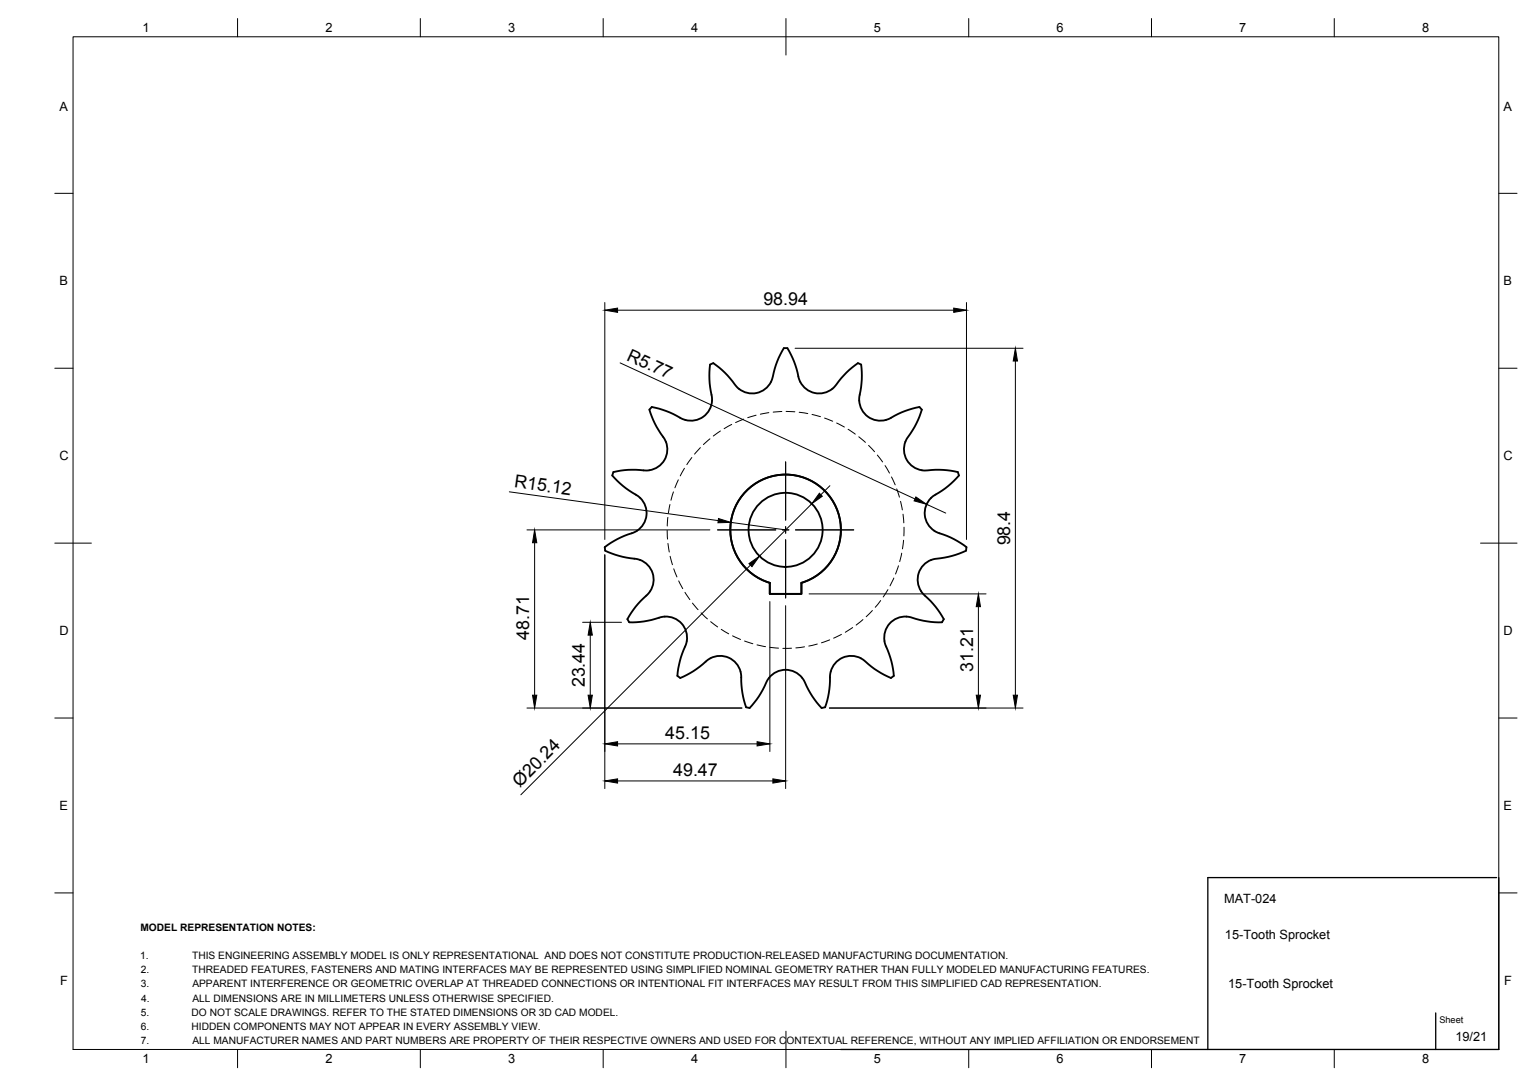
ISO-10303-21;
HEADER;
/* Generated by software containing ST-Developer
 * from STEP Tools, Inc. (www.steptools.com) 
 */

FILE_DESCRIPTION(
/* description */ ('STEP AP214'),
/* implementation_level */ '2;1');

FILE_NAME(
/* name */ '15-Tooth Sprocket.step',
/* time_stamp */ '2026-11-14T06:34:07-08:00',
/* author */ (''),
/* organization */ (''),
/* preprocessor_version */ 'ST-DEVELOPER v20.2',
/* originating_system */ 'Autodesk Translation Framework v15.17.0.0',
/* authorisation */ '');

FILE_SCHEMA (('AUTOMOTIVE_DESIGN { 1 0 10303 214 3 1 1 }'));
ENDSEC;

DATA;
#10=MECHANICAL_DESIGN_GEOMETRIC_PRESENTATION_REPRESENTATION('',(#7279,#7280),#310623);
#4024=TOROIDAL_SURFACE('',#103341,32.976,0.576);
#4025=TOROIDAL_SURFACE('',#103396,40.6764810164406,18.288);
#4026=TOROIDAL_SURFACE('',#103398,40.6764810164406,18.288);
#4027=TOROIDAL_SURFACE('',#103400,40.6764810164406,18.288);
#4028=TOROIDAL_SURFACE('',#103402,40.6764810164406,18.288);
#4029=TOROIDAL_SURFACE('',#103404,40.6764810164406,18.288);
#4030=TOROIDAL_SURFACE('',#103406,40.6764810164406,18.288);
#4031=TOROIDAL_SURFACE('',#103408,40.6764810164406,18.288);
#4032=TOROIDAL_SURFACE('',#103410,40.6764810164406,18.288);
#4033=TOROIDAL_SURFACE('',#103412,40.6764810164406,18.288);
#4034=TOROIDAL_SURFACE('',#103414,40.6764810164406,18.288);
#4035=TOROIDAL_SURFACE('',#103416,40.6764810164406,18.288);
#4036=TOROIDAL_SURFACE('',#103418,40.6764810164406,18.288);
#4037=TOROIDAL_SURFACE('',#103420,40.6764810164406,18.288);
#4038=TOROIDAL_SURFACE('',#103422,40.6764810164406,18.288);
#4039=TOROIDAL_SURFACE('',#103452,40.6764810164406,18.288);
#4040=TOROIDAL_SURFACE('',#103454,40.6764810164406,18.288);
#4041=TOROIDAL_SURFACE('',#103456,40.6764810164406,18.288);
#4042=TOROIDAL_SURFACE('',#103458,40.6764810164406,18.288);
#4043=TOROIDAL_SURFACE('',#103460,40.6764810164406,18.288);
#4044=TOROIDAL_SURFACE('',#103462,40.6764810164406,18.288);
#4045=TOROIDAL_SURFACE('',#103464,40.6764810164406,18.288);
#4046=TOROIDAL_SURFACE('',#103466,40.6764810164406,18.288);
#4047=TOROIDAL_SURFACE('',#103468,40.6764810164406,18.288);
#4048=TOROIDAL_SURFACE('',#103470,40.6764810164406,18.288);
#4049=TOROIDAL_SURFACE('',#103472,40.6764810164406,18.288);
#4050=TOROIDAL_SURFACE('',#103474,40.6764810164406,18.288);
#4051=TOROIDAL_SURFACE('',#103476,40.6764810164406,18.288);
#4052=TOROIDAL_SURFACE('',#103478,40.6764810164406,18.288);
#4053=TOROIDAL_SURFACE('',#103480,40.6764810164406,18.288);
#4054=TOROIDAL_SURFACE('',#103484,40.6764810164406,18.288);
#6306=B_SPLINE_CURVE_WITH_KNOTS('',3,(#271237,#271238,#271239,#271240,#271241,
#271242,#271243,#271244),.UNSPECIFIED.,.F.,.F.,(4,2,2,4),(-8.98049293427854,
-8.97889171867458,-8.34884827602697,-8.12983481855878),.UNSPECIFIED.);
#6307=B_SPLINE_CURVE_WITH_KNOTS('',3,(#271248,#271249,#271250,#271251,#271252,
#271253),.UNSPECIFIED.,.F.,.F.,(4,2,4),(-2.68771546706156,-2.29799156778152,
-1.97285776109994),.UNSPECIFIED.);
#6308=B_SPLINE_CURVE_WITH_KNOTS('',3,(#271258,#271259,#271260,#271261,#271262,
#271263),.UNSPECIFIED.,.F.,.F.,(4,2,4),(0.518273427329016,0.647448708132802,
0.677306880099543),.UNSPECIFIED.);
#6309=B_SPLINE_CURVE_WITH_KNOTS('',3,(#271267,#271268,#271269,#271270),
 .UNSPECIFIED.,.F.,.F.,(4,4),(1.16920248436213,1.3284621703947),
 .UNSPECIFIED.);
#6310=B_SPLINE_CURVE_WITH_KNOTS('',3,(#271274,#271275,#271276,#271277,#271278,
#271279),.UNSPECIFIED.,.F.,.F.,(4,2,4),(2.36444145730686,2.40335316097516,
2.52343865872206),.UNSPECIFIED.);
#6311=B_SPLINE_CURVE_WITH_KNOTS('',3,(#271283,#271284,#271285,#271286,#271287,
#271288),.UNSPECIFIED.,.F.,.F.,(4,2,4),(3.01719559991105,3.07732160469005,
3.17624638273508),.UNSPECIFIED.);
#6312=B_SPLINE_CURVE_WITH_KNOTS('',3,(#271295,#271296,#271297,#271298,#271299,
#271300),.UNSPECIFIED.,.F.,.F.,(4,2,4),(0.51827342732949,0.647448708132718,
0.677306880099455),.UNSPECIFIED.);
#6313=B_SPLINE_CURVE_WITH_KNOTS('',3,(#271304,#271305,#271306,#271307),
 .UNSPECIFIED.,.F.,.F.,(4,4),(1.16920248460095,1.3284621706712),
 .UNSPECIFIED.);
#6314=B_SPLINE_CURVE_WITH_KNOTS('',3,(#271311,#271312,#271313,#271314,#271315,
#271316),.UNSPECIFIED.,.F.,.F.,(4,2,4),(2.36444145785531,2.40335316153482,
2.5234386593167),.UNSPECIFIED.);
#6315=B_SPLINE_CURVE_WITH_KNOTS('',3,(#271319,#271320,#271321,#271322,#271323,
#271324),.UNSPECIFIED.,.F.,.F.,(4,2,4),(3.01719559991067,3.07732160468965,
3.17624638273467),.UNSPECIFIED.);
#6316=B_SPLINE_CURVE_WITH_KNOTS('',3,(#271330,#271331,#271332,#271333,#271334,
#271335),.UNSPECIFIED.,.F.,.F.,(4,2,4),(0.51827342732973,0.647448708133012,
0.677306880099766),.UNSPECIFIED.);
#6317=B_SPLINE_CURVE_WITH_KNOTS('',3,(#271339,#271340,#271341,#271342),
 .UNSPECIFIED.,.F.,.F.,(4,4),(1.16920248436227,1.32846217039502),
 .UNSPECIFIED.);
#6318=B_SPLINE_CURVE_WITH_KNOTS('',3,(#271346,#271347,#271348,#271349,#271350,
#271351),.UNSPECIFIED.,.F.,.F.,(4,2,4),(2.36444145730766,2.40335316097597,
2.523438658723),.UNSPECIFIED.);
#6319=B_SPLINE_CURVE_WITH_KNOTS('',3,(#271354,#271355,#271356,#271357,#271358,
#271359),.UNSPECIFIED.,.F.,.F.,(4,2,4),(3.0171955999124,3.07732160469143,
3.1762463827365),.UNSPECIFIED.);
#6320=B_SPLINE_CURVE_WITH_KNOTS('',3,(#271363,#271364,#271365,#271366,#271367,
#271368),.UNSPECIFIED.,.F.,.F.,(4,2,4),(3.01719559991218,3.07732160469121,
3.17624638273563),.UNSPECIFIED.);
#6321=B_SPLINE_CURVE_WITH_KNOTS('',3,(#271372,#271373,#271374,#271375,#271376,
#271377),.UNSPECIFIED.,.F.,.F.,(4,2,4),(0.518273427329665,0.647448708132928,
0.677306880099671),.UNSPECIFIED.);
#6322=B_SPLINE_CURVE_WITH_KNOTS('',3,(#271381,#271382,#271383,#271384),
 .UNSPECIFIED.,.F.,.F.,(4,4),(1.1692024843613,1.32846217039385),
 .UNSPECIFIED.);
#6323=B_SPLINE_CURVE_WITH_KNOTS('',3,(#271388,#271389,#271390,#271391,#271392,
#271393),.UNSPECIFIED.,.F.,.F.,(4,2,4),(2.36444145730499,2.40335316097287,
2.52343865871962),.UNSPECIFIED.);
#6324=B_SPLINE_CURVE_WITH_KNOTS('',3,(#271400,#271401,#271402,#271403,#271404,
#271405),.UNSPECIFIED.,.F.,.F.,(4,2,4),(0.518273427329571,0.647448708132802,
0.677306880099541),.UNSPECIFIED.);
#6325=B_SPLINE_CURVE_WITH_KNOTS('',3,(#271409,#271410,#271411,#271412),
 .UNSPECIFIED.,.F.,.F.,(4,4),(1.16920248412223,1.32846217011725),
 .UNSPECIFIED.);
#6326=B_SPLINE_CURVE_WITH_KNOTS('',3,(#271416,#271417,#271418,#271419,#271420,
#271421),.UNSPECIFIED.,.F.,.F.,(4,2,4),(2.3644414567562,2.40335316041326,
2.52343865812509),.UNSPECIFIED.);
#6327=B_SPLINE_CURVE_WITH_KNOTS('',3,(#271424,#271425,#271426,#271427,#271428,
#271429),.UNSPECIFIED.,.F.,.F.,(4,2,4),(3.01719559991075,3.07732160468976,
3.17624638273476),.UNSPECIFIED.);
#6328=B_SPLINE_CURVE_WITH_KNOTS('',3,(#271435,#271436,#271437,#271438,#271439,
#271440),.UNSPECIFIED.,.F.,.F.,(4,2,4),(0.518273427329574,0.647448708132822,
0.677306880099564),.UNSPECIFIED.);
#6329=B_SPLINE_CURVE_WITH_KNOTS('',3,(#271444,#271445,#271446,#271447),
 .UNSPECIFIED.,.F.,.F.,(4,4),(1.16920248436231,1.32846217039508),
 .UNSPECIFIED.);
#6330=B_SPLINE_CURVE_WITH_KNOTS('',3,(#271451,#271452,#271453,#271454,#271455,
#271456),.UNSPECIFIED.,.F.,.F.,(4,2,4),(2.3644414573074,2.40335316097572,
2.52343865872264),.UNSPECIFIED.);
#6331=B_SPLINE_CURVE_WITH_KNOTS('',3,(#271459,#271460,#271461,#271462,#271463,
#271464),.UNSPECIFIED.,.F.,.F.,(4,2,4),(3.01719559991156,3.07732160469059,
3.17624638273566),.UNSPECIFIED.);
#6332=B_SPLINE_CURVE_WITH_KNOTS('',3,(#271468,#271469,#271470,#271471,#271472,
#271473),.UNSPECIFIED.,.F.,.F.,(4,2,4),(-2.68771546706066,-2.29799156778083,
-1.9728577610994),.UNSPECIFIED.);
#6333=B_SPLINE_CURVE_WITH_KNOTS('',3,(#271477,#271478,#271479,#271480,#271481,
#271482,#271483,#271484),.UNSPECIFIED.,.F.,.F.,(4,2,2,4),(-8.98049293427925,
-8.97889171867529,-8.34884827602781,-8.12983481855968),.UNSPECIFIED.);
#6334=B_SPLINE_CURVE_WITH_KNOTS('',3,(#271552,#271553,#271554,#271555,#271556,
#271557,#271558,#271559),.UNSPECIFIED.,.F.,.F.,(4,2,2,4),(-8.98049293427854,
-8.97889171867458,-8.34884827602725,-8.12983481855919),.UNSPECIFIED.);
#6335=B_SPLINE_CURVE_WITH_KNOTS('',3,(#271563,#271564,#271565,#271566,#271567,
#271568),.UNSPECIFIED.,.F.,.F.,(4,2,4),(-2.68771546706143,-2.29799156778143,
-1.97285776109989),.UNSPECIFIED.);
#6336=B_SPLINE_CURVE_WITH_KNOTS('',3,(#271569,#271570,#271571,#271572,#271573,
#271574),.UNSPECIFIED.,.F.,.F.,(4,2,4),(0.51827342732961,0.64744870813287,
0.677306880099612),.UNSPECIFIED.);
#6337=B_SPLINE_CURVE_WITH_KNOTS('',3,(#271575,#271576,#271577,#271578,#271579,
#271580),.UNSPECIFIED.,.F.,.F.,(4,2,4),(3.0171955999114,3.07732160469042,
3.17624638273548),.UNSPECIFIED.);
#6338=B_SPLINE_CURVE_WITH_KNOTS('',3,(#271583,#271584,#271585,#271586,#271587,
#271588),.UNSPECIFIED.,.F.,.F.,(4,2,4),(0.518273427329597,0.647448708132832,
0.677306880099573),.UNSPECIFIED.);
#6339=B_SPLINE_CURVE_WITH_KNOTS('',3,(#271590,#271591,#271592,#271593,#271594,
#271595),.UNSPECIFIED.,.F.,.F.,(4,2,4),(3.01719559990933,3.07732160468829,
3.17624638273323),.UNSPECIFIED.);
#6340=B_SPLINE_CURVE_WITH_KNOTS('',3,(#271597,#271598,#271599,#271600,#271601,
#271602,#271603,#271604),.UNSPECIFIED.,.F.,.F.,(4,2,2,4),(-8.98049293427795,
-8.97889171867398,-8.3488482760265,-8.12983481855838),.UNSPECIFIED.);
#6341=B_SPLINE_CURVE_WITH_KNOTS('',3,(#271607,#271608,#271609,#271610,#271611,
#271612),.UNSPECIFIED.,.F.,.F.,(4,2,4),(-2.6877154670615,-2.29799156778146,
-1.97285776109988),.UNSPECIFIED.);
#6342=B_SPLINE_CURVE_WITH_KNOTS('',3,(#271615,#271616,#271617,#271618,#271619,
#271620),.UNSPECIFIED.,.F.,.F.,(4,2,4),(0.518273427329312,0.647448708132468,
0.677306880099178),.UNSPECIFIED.);
#6343=B_SPLINE_CURVE_WITH_KNOTS('',3,(#271622,#271623,#271624,#271625,#271626,
#271627),.UNSPECIFIED.,.F.,.F.,(4,2,4),(3.0171955999108,3.0773216046898,
3.1762463827348),.UNSPECIFIED.);
#6344=B_SPLINE_CURVE_WITH_KNOTS('',3,(#271629,#271630,#271631,#271632,#271633,
#271634,#271635,#271636),.UNSPECIFIED.,.F.,.F.,(4,2,2,4),(-8.98049293427752,
-8.97889171867356,-8.34884827602617,-8.12983481855807),.UNSPECIFIED.);
#6345=B_SPLINE_CURVE_WITH_KNOTS('',3,(#271639,#271640,#271641,#271642,#271643,
#271644),.UNSPECIFIED.,.F.,.F.,(4,2,4),(-2.68771546706155,-2.29799156778148,
-1.9728577610999),.UNSPECIFIED.);
#6346=B_SPLINE_CURVE_WITH_KNOTS('',3,(#271647,#271648,#271649,#271650,#271651,
#271652),.UNSPECIFIED.,.F.,.F.,(4,2,4),(0.518273427329541,0.647448708132767,
0.6773068800995),.UNSPECIFIED.);
#6347=B_SPLINE_CURVE_WITH_KNOTS('',3,(#271654,#271655,#271656,#271657,#271658,
#271659),.UNSPECIFIED.,.F.,.F.,(4,2,4),(3.01719559991074,3.07732160468976,
3.17624638273482),.UNSPECIFIED.);
#6348=B_SPLINE_CURVE_WITH_KNOTS('',3,(#271661,#271662,#271663,#271664,#271665,
#271666,#271667,#271668),.UNSPECIFIED.,.F.,.F.,(4,2,2,4),(-8.98049293427772,
-8.97889171867376,-8.34884827602598,-8.12983481855773),.UNSPECIFIED.);
#6349=B_SPLINE_CURVE_WITH_KNOTS('',3,(#271671,#271672,#271673,#271674,#271675,
#271676),.UNSPECIFIED.,.F.,.F.,(4,2,4),(-2.68771546706066,-2.29799156778086,
-1.97285776109946),.UNSPECIFIED.);
#6350=B_SPLINE_CURVE_WITH_KNOTS('',3,(#271681,#271682,#271683,#271684,#271685,
#271686),.UNSPECIFIED.,.F.,.F.,(4,2,4),(-2.68771546706142,-2.29799156778141,
-1.97285776109986),.UNSPECIFIED.);
#6351=B_SPLINE_CURVE_WITH_KNOTS('',3,(#271687,#271688,#271689,#271690,#271691,
#271692),.UNSPECIFIED.,.F.,.F.,(4,2,4),(0.518273427329233,0.647448708132411,
0.677306880099119),.UNSPECIFIED.);
#6352=B_SPLINE_CURVE_WITH_KNOTS('',3,(#271693,#271694,#271695,#271696,#271697,
#271698),.UNSPECIFIED.,.F.,.F.,(4,2,4),(3.01719559991029,3.0773216046893,
3.17624638273431),.UNSPECIFIED.);
#6353=B_SPLINE_CURVE_WITH_KNOTS('',3,(#271701,#271702,#271703,#271704,#271705,
#271706),.UNSPECIFIED.,.F.,.F.,(4,2,4),(0.518273427329369,0.647448708132555,
0.677306880099271),.UNSPECIFIED.);
#6354=B_SPLINE_CURVE_WITH_KNOTS('',3,(#271708,#271709,#271710,#271711,#271712,
#271713),.UNSPECIFIED.,.F.,.F.,(4,2,4),(3.01719559991216,3.07732160469119,
3.17624638273627),.UNSPECIFIED.);
#6355=B_SPLINE_CURVE_WITH_KNOTS('',3,(#271715,#271716,#271717,#271718,#271719,
#271720,#271721,#271722),.UNSPECIFIED.,.F.,.F.,(4,2,2,4),(-8.98049293427722,
-8.97889171867326,-8.34884827602583,-8.1298348185577),.UNSPECIFIED.);
#6356=B_SPLINE_CURVE_WITH_KNOTS('',3,(#271725,#271726,#271727,#271728,#271729,
#271730),.UNSPECIFIED.,.F.,.F.,(4,2,4),(-2.68771546706111,-2.29799156778117,
-1.97285776109968),.UNSPECIFIED.);
#6357=B_SPLINE_CURVE_WITH_KNOTS('',3,(#271734,#271735,#271736,#271737,#271738,
#271739,#271740,#271741),.UNSPECIFIED.,.F.,.F.,(4,2,2,4),(-8.98049293427961,
-8.97889171867565,-8.34884827602804,-8.12983481855986),.UNSPECIFIED.);
#6358=B_SPLINE_CURVE_WITH_KNOTS('',3,(#271745,#271746,#271747,#271748,#271749,
#271750),.UNSPECIFIED.,.F.,.F.,(4,2,4),(-2.68771546706186,-2.29799156778171,
-1.97285776110007),.UNSPECIFIED.);
#6359=B_SPLINE_CURVE_WITH_KNOTS('',3,(#271751,#271752,#271753,#271754,#271755,
#271756),.UNSPECIFIED.,.F.,.F.,(4,2,4),(0.51827342732934,0.647448708132526,
0.677306880099254),.UNSPECIFIED.);
#6360=B_SPLINE_CURVE_WITH_KNOTS('',3,(#271757,#271758,#271759,#271760,#271761,
#271762),.UNSPECIFIED.,.F.,.F.,(4,2,4),(3.01719559990916,3.07732160468812,
3.17624638273306),.UNSPECIFIED.);
#6361=B_SPLINE_CURVE_WITH_KNOTS('',3,(#271765,#271766,#271767,#271768,#271769,
#271770,#271771,#271772),.UNSPECIFIED.,.F.,.F.,(4,2,2,4),(-8.98049293427778,
-8.97889171867381,-8.34884827602637,-8.12983481855824),.UNSPECIFIED.);
#6362=B_SPLINE_CURVE_WITH_KNOTS('',3,(#271775,#271776,#271777,#271778,#271779,
#271780),.UNSPECIFIED.,.F.,.F.,(4,2,4),(-2.68771546706139,-2.29799156778137,
-1.97285776109982),.UNSPECIFIED.);
#6363=B_SPLINE_CURVE_WITH_KNOTS('',3,(#271783,#271784,#271785,#271786,#271787,
#271788),.UNSPECIFIED.,.F.,.F.,(4,2,4),(3.01719559990971,3.07732160468868,
3.17624638273366),.UNSPECIFIED.);
#6364=B_SPLINE_CURVE_WITH_KNOTS('',3,(#271790,#271791,#271792,#271793,#271794,
#271795,#271796,#271797),.UNSPECIFIED.,.F.,.F.,(4,2,2,4),(-8.98049293427817,
-8.97889171867421,-8.34884827602685,-8.12983481855876),.UNSPECIFIED.);
#6365=B_SPLINE_CURVE_WITH_KNOTS('',3,(#271800,#271801,#271802,#271803,#271804,
#271805),.UNSPECIFIED.,.F.,.F.,(4,2,4),(-2.68771546706148,-2.29799156778145,
-1.97285776109989),.UNSPECIFIED.);
#6366=B_SPLINE_CURVE_WITH_KNOTS('',3,(#271808,#271809,#271810,#271811,#271812,
#271813,#271814,#271815),.UNSPECIFIED.,.F.,.F.,(4,2,2,4),(-8.98049293427992,
-8.97889171867596,-8.34884827602816,-8.12983481855992),.UNSPECIFIED.);
#6367=B_SPLINE_CURVE_WITH_KNOTS('',3,(#271818,#271819,#271820,#271821,#271822,
#271823),.UNSPECIFIED.,.F.,.F.,(4,2,4),(-2.68771546706129,-2.29799156778129,
-1.97285776109976),.UNSPECIFIED.);
#6368=B_SPLINE_CURVE_WITH_KNOTS('',3,(#271826,#271827,#271828,#271829,#271830,
#271831,#271832,#271833),.UNSPECIFIED.,.F.,.F.,(4,2,2,4),(-8.98049293428024,
-8.97889171867627,-8.34884827602869,-8.12983481856052),.UNSPECIFIED.);
#6369=B_SPLINE_CURVE_WITH_KNOTS('',3,(#271836,#271837,#271838,#271839,#271840,
#271841),.UNSPECIFIED.,.F.,.F.,(4,2,4),(-2.68771546706172,-2.29799156778164,
-1.97285776110006),.UNSPECIFIED.);
#6370=B_SPLINE_CURVE_WITH_KNOTS('',3,(#271844,#271845,#271846,#271847,#271848,
#271849,#271850,#271851),.UNSPECIFIED.,.F.,.F.,(4,2,2,4),(-8.98049293427857,
-8.97889171867461,-8.34884827602675,-8.12983481855846),.UNSPECIFIED.);
#6371=B_SPLINE_CURVE_WITH_KNOTS('',3,(#271854,#271855,#271856,#271857,#271858,
#271859),.UNSPECIFIED.,.F.,.F.,(4,2,4),(-2.68771546706135,-2.29799156778136,
-1.97285776109983),.UNSPECIFIED.);
#6372=B_SPLINE_CURVE_WITH_KNOTS('',3,(#271862,#271863,#271864,#271865,#271866,
#271867,#271868,#271869),.UNSPECIFIED.,.F.,.F.,(4,2,2,4),(-8.98049293428122,
-8.97889171867726,-8.34884827602979,-8.12983481856169),.UNSPECIFIED.);
#6373=B_SPLINE_CURVE_WITH_KNOTS('',3,(#271873,#271874,#271875,#271876,#271877,
#271878),.UNSPECIFIED.,.F.,.F.,(4,2,4),(-2.68771546706168,-2.29799156778158,
-1.97285776109999),.UNSPECIFIED.);
#6374=B_SPLINE_CURVE_WITH_KNOTS('',3,(#271879,#271880,#271881,#271882,#271883,
#271884),.UNSPECIFIED.,.F.,.F.,(4,2,4),(0.518273427329314,0.647448708132495,
0.677306880099206),.UNSPECIFIED.);
#6375=B_SPLINE_CURVE_WITH_KNOTS('',3,(#271887,#271888,#271889,#271890,#271891,
#271892,#271893,#271894),.UNSPECIFIED.,.F.,.F.,(4,2,2,4),(-8.98049293427992,
-8.97889171867595,-8.34884827602839,-8.12983481856025),.UNSPECIFIED.);
#6376=B_SPLINE_CURVE_WITH_KNOTS('',3,(#271897,#271898,#271899,#271900,#271901,
#271902),.UNSPECIFIED.,.F.,.F.,(4,2,4),(-2.68771546706109,-2.29799156778117,
-1.97285776109969),.UNSPECIFIED.);
#6377=B_SPLINE_CURVE_WITH_KNOTS('',3,(#271987,#271988,#271989,#271990,#271991,
#271992),.UNSPECIFIED.,.F.,.F.,(4,2,4),(-2.68771546706178,-2.29799156778168,
-1.97285776110008),.UNSPECIFIED.);
#6378=B_SPLINE_CURVE_WITH_KNOTS('',3,(#271994,#271995,#271996,#271997,#271998,
#271999),.UNSPECIFIED.,.F.,.F.,(4,2,4),(2.36444145730966,2.403353160978,
2.52343865872509),.UNSPECIFIED.);
#6379=B_SPLINE_CURVE_WITH_KNOTS('',3,(#272003,#272004,#272005,#272006),
 .UNSPECIFIED.,.F.,.F.,(4,4),(1.16920248436245,1.32846217039523),
 .UNSPECIFIED.);
#6380=B_SPLINE_CURVE_WITH_KNOTS('',3,(#272007,#272008,#272009,#272010,#272011,
#272012,#272013,#272014),.UNSPECIFIED.,.F.,.F.,(4,2,2,4),(-8.98049293428071,
-8.97889171867675,-8.34884827602921,-8.12983481856106),.UNSPECIFIED.);
#6381=B_SPLINE_CURVE_WITH_KNOTS('',3,(#272018,#272019,#272020,#272021),
 .UNSPECIFIED.,.F.,.F.,(4,4),(1.16920248436348,1.32846217039639),
 .UNSPECIFIED.);
#6382=B_SPLINE_CURVE_WITH_KNOTS('',3,(#272022,#272023,#272024,#272025,#272026,
#272027,#272028,#272029),.UNSPECIFIED.,.F.,.F.,(4,2,2,4),(-8.98049293427966,
-8.97889171867569,-8.34884827602823,-8.12983481856012),.UNSPECIFIED.);
#6383=B_SPLINE_CURVE_WITH_KNOTS('',3,(#272031,#272032,#272033,#272034,#272035,
#272036),.UNSPECIFIED.,.F.,.F.,(4,2,4),(-2.68771546706079,-2.29799156778091,
-1.97285776109946),.UNSPECIFIED.);
#6384=B_SPLINE_CURVE_WITH_KNOTS('',3,(#272038,#272039,#272040,#272041,#272042,
#272043),.UNSPECIFIED.,.F.,.F.,(4,2,4),(2.36444145731017,2.40335316097854,
2.52343865872566),.UNSPECIFIED.);
#6385=B_SPLINE_CURVE_WITH_KNOTS('',3,(#272048,#272049,#272050,#272051),
 .UNSPECIFIED.,.F.,.F.,(4,4),(1.16920248436344,1.32846217039637),
 .UNSPECIFIED.);
#6386=B_SPLINE_CURVE_WITH_KNOTS('',3,(#272052,#272053,#272054,#272055,#272056,
#272057,#272058,#272059),.UNSPECIFIED.,.F.,.F.,(4,2,2,4),(-8.98049293427945,
-8.97889171867549,-8.34884827602783,-8.12983481855963),.UNSPECIFIED.);
#6387=B_SPLINE_CURVE_WITH_KNOTS('',3,(#272061,#272062,#272063,#272064,#272065,
#272066),.UNSPECIFIED.,.F.,.F.,(4,2,4),(-2.68771546706122,-2.29799156778128,
-1.97285776109977),.UNSPECIFIED.);
#6388=B_SPLINE_CURVE_WITH_KNOTS('',3,(#272068,#272069,#272070,#272071,#272072,
#272073),.UNSPECIFIED.,.F.,.F.,(4,2,4),(2.36444145675313,2.40335316041008,
2.52343865812168),.UNSPECIFIED.);
#6389=B_SPLINE_CURVE_WITH_KNOTS('',3,(#272078,#272079,#272080,#272081),
 .UNSPECIFIED.,.F.,.F.,(4,4),(1.16920248412103,1.32846217011589),
 .UNSPECIFIED.);
#6390=B_SPLINE_CURVE_WITH_KNOTS('',3,(#272082,#272083,#272084,#272085,#272086,
#272087,#272088,#272089),.UNSPECIFIED.,.F.,.F.,(4,2,2,4),(-8.98049293427762,
-8.97889171867365,-8.34884827602598,-8.12983481855776),.UNSPECIFIED.);
#6391=B_SPLINE_CURVE_WITH_KNOTS('',3,(#272091,#272092,#272093,#272094,#272095,
#272096),.UNSPECIFIED.,.F.,.F.,(4,2,4),(-2.68771546706239,-2.29799156778215,
-1.97285776110044),.UNSPECIFIED.);
#6392=B_SPLINE_CURVE_WITH_KNOTS('',3,(#272098,#272099,#272100,#272101,#272102,
#272103),.UNSPECIFIED.,.F.,.F.,(4,2,4),(2.36444145730695,2.40335316097526,
2.5234386587222),.UNSPECIFIED.);
#6393=B_SPLINE_CURVE_WITH_KNOTS('',3,(#272107,#272108,#272109,#272110,#272111,
#272112),.UNSPECIFIED.,.F.,.F.,(4,2,4),(2.36444145785125,2.4033531615307,
2.52343865931237),.UNSPECIFIED.);
#6394=B_SPLINE_CURVE_WITH_KNOTS('',3,(#272116,#272117,#272118,#272119),
 .UNSPECIFIED.,.F.,.F.,(4,4),(1.16920248436207,1.3284621703948),
 .UNSPECIFIED.);
#6395=B_SPLINE_CURVE_WITH_KNOTS('',3,(#272120,#272121,#272122,#272123,#272124,
#272125,#272126,#272127),.UNSPECIFIED.,.F.,.F.,(4,2,2,4),(-8.98049293427944,
-8.97889171867548,-8.34884827602771,-8.12983481855948),.UNSPECIFIED.);
#6396=B_SPLINE_CURVE_WITH_KNOTS('',3,(#272131,#272132,#272133,#272134),
 .UNSPECIFIED.,.F.,.F.,(4,4),(1.16920248459907,1.32846217066903),
 .UNSPECIFIED.);
#6397=B_SPLINE_CURVE_WITH_KNOTS('',3,(#272135,#272136,#272137,#272138,#272139,
#272140,#272141,#272142),.UNSPECIFIED.,.F.,.F.,(4,2,2,4),(-8.98049293428055,
-8.97889171867659,-8.34884827602886,-8.12983481856065),.UNSPECIFIED.);
#6398=B_SPLINE_CURVE_WITH_KNOTS('',3,(#272144,#272145,#272146,#272147,#272148,
#272149),.UNSPECIFIED.,.F.,.F.,(4,2,4),(-2.68771546706087,-2.297991567781,
-1.97285776109955),.UNSPECIFIED.);
#6399=B_SPLINE_CURVE_WITH_KNOTS('',3,(#272151,#272152,#272153,#272154,#272155,
#272156),.UNSPECIFIED.,.F.,.F.,(4,2,4),(2.36444145730775,2.4033531609761,
2.5234386587231),.UNSPECIFIED.);
#6400=B_SPLINE_CURVE_WITH_KNOTS('',3,(#272160,#272161,#272162,#272163,#272164,
#272165),.UNSPECIFIED.,.F.,.F.,(4,2,4),(-2.68771546706131,-2.29799156778135,
-1.97285776109984),.UNSPECIFIED.);
#6401=B_SPLINE_CURVE_WITH_KNOTS('',3,(#272167,#272168,#272169,#272170,#272171,
#272172),.UNSPECIFIED.,.F.,.F.,(4,2,4),(2.36444145730746,2.40335316097579,
2.52343865872281),.UNSPECIFIED.);
#6402=B_SPLINE_CURVE_WITH_KNOTS('',3,(#272176,#272177,#272178,#272179),
 .UNSPECIFIED.,.F.,.F.,(4,4),(1.16920248412219,1.32846217011718),
 .UNSPECIFIED.);
#6403=B_SPLINE_CURVE_WITH_KNOTS('',3,(#272180,#272181,#272182,#272183,#272184,
#272185,#272186,#272187),.UNSPECIFIED.,.F.,.F.,(4,2,2,4),(-8.98049293428066,
-8.9788917186767,-8.34884827602938,-8.12983481856134),.UNSPECIFIED.);
#6404=B_SPLINE_CURVE_WITH_KNOTS('',3,(#272189,#272190,#272191,#272192,#272193,
#272194),.UNSPECIFIED.,.F.,.F.,(4,2,4),(-2.68771546706095,-2.29799156778107,
-1.97285776109961),.UNSPECIFIED.);
#6405=B_SPLINE_CURVE_WITH_KNOTS('',3,(#272196,#272197,#272198,#272199,#272200,
#272201,#272202,#272203),.UNSPECIFIED.,.F.,.F.,(4,2,2,4),(-8.98049293427952,
-8.97889171867556,-8.34884827602786,-8.12983481855966),.UNSPECIFIED.);
#6406=B_SPLINE_CURVE_WITH_KNOTS('',3,(#272205,#272206,#272207,#272208,#272209,
#272210,#272211,#272212),.UNSPECIFIED.,.F.,.F.,(4,2,2,4),(-8.98049293428018,
-8.97889171867621,-8.34884827602859,-8.12983481856041),.UNSPECIFIED.);
#6407=B_SPLINE_CURVE_WITH_KNOTS('',3,(#272214,#272215,#272216,#272217,#272218,
#272219),.UNSPECIFIED.,.F.,.F.,(4,2,4),(-2.68771546706135,-2.29799156778134,
-1.9728577610998),.UNSPECIFIED.);
#6408=B_SPLINE_CURVE_WITH_KNOTS('',3,(#272221,#272222,#272223,#272224,#272225,
#272226),.UNSPECIFIED.,.F.,.F.,(4,2,4),(2.36444145675532,2.40335316041232,
2.52343865812401),.UNSPECIFIED.);
#6409=B_SPLINE_CURVE_WITH_KNOTS('',3,(#272229,#272230,#272231,#272232,#272233,
#272234),.UNSPECIFIED.,.F.,.F.,(4,2,4),(-2.68771546706153,-2.2979915677815,
-1.97285776109994),.UNSPECIFIED.);
#6410=B_SPLINE_CURVE_WITH_KNOTS('',3,(#272236,#272237,#272238,#272239,#272240,
#272241,#272242,#272243),.UNSPECIFIED.,.F.,.F.,(4,2,2,4),(-8.98049293427927,
-8.97889171867531,-8.34884827602772,-8.12983481855955),.UNSPECIFIED.);
#6411=B_SPLINE_CURVE_WITH_KNOTS('',3,(#272245,#272246,#272247,#272248,#272249,
#272250),.UNSPECIFIED.,.F.,.F.,(4,2,4),(-2.68771546706105,-2.29799156778115,
-1.97285776109967),.UNSPECIFIED.);
#6412=B_SPLINE_CURVE_WITH_KNOTS('',3,(#272252,#272253,#272254,#272255,#272256,
#272257,#272258,#272259),.UNSPECIFIED.,.F.,.F.,(4,2,2,4),(-8.98049293428103,
-8.97889171867707,-8.34884827602985,-8.12983481856184),.UNSPECIFIED.);
#6413=B_SPLINE_CURVE_WITH_KNOTS('',3,(#272261,#272262,#272263,#272264,#272265,
#272266,#272267,#272268),.UNSPECIFIED.,.F.,.F.,(4,2,2,4),(-8.98049293428005,
-8.97889171867609,-8.34884827602866,-8.12983481856055),.UNSPECIFIED.);
#6414=B_SPLINE_CURVE_WITH_KNOTS('',3,(#272269,#272270,#272271,#272272,#272273,
#272274),.UNSPECIFIED.,.F.,.F.,(4,2,4),(-2.68771546706036,-2.29799156778066,
-1.97285776109931),.UNSPECIFIED.);
#6415=B_SPLINE_CURVE_WITH_KNOTS('',3,(#272277,#272278,#272279,#272280,#272281,
#272282),.UNSPECIFIED.,.F.,.F.,(4,2,4),(-2.68771546706178,-2.2979915677817,
-1.9728577611001),.UNSPECIFIED.);
#6416=B_SPLINE_CURVE_WITH_KNOTS('',3,(#272286,#272287,#272288,#272289),
 .UNSPECIFIED.,.F.,.F.,(4,4),(1.16920248412169,1.32846217011663),
 .UNSPECIFIED.);
#6417=B_SPLINE_CURVE_WITH_KNOTS('',3,(#272290,#272291,#272292,#272293,#272294,
#272295,#272296,#272297),.UNSPECIFIED.,.F.,.F.,(4,2,2,4),(-8.98049293427827,
-8.9788917186743,-8.34884827602666,-8.12983481855847),.UNSPECIFIED.);
#6418=B_SPLINE_CURVE_WITH_KNOTS('',3,(#272299,#272300,#272301,#272302,#272303,
#272304,#272305,#272306),.UNSPECIFIED.,.F.,.F.,(4,2,2,4),(-8.98049293428091,
-8.97889171867695,-8.34884827602936,-8.12983481856121),.UNSPECIFIED.);
#6419=B_SPLINE_CURVE_WITH_KNOTS('',3,(#272307,#272308,#272309,#272310,#272311,
#272312),.UNSPECIFIED.,.F.,.F.,(4,2,4),(-2.68771546706137,-2.29799156778137,
-1.97285776109986),.UNSPECIFIED.);
#6420=B_SPLINE_CURVE_WITH_KNOTS('',3,(#272315,#272316,#272317,#272318,#272319,
#272320),.UNSPECIFIED.,.F.,.F.,(4,2,4),(0.518273427329387,0.647448708132598,
0.677306880099315),.UNSPECIFIED.);
#6421=B_SPLINE_CURVE_WITH_KNOTS('',3,(#272322,#272323,#272324,#272325,#272326,
#272327),.UNSPECIFIED.,.F.,.F.,(4,2,4),(3.01719559990939,3.07732160468838,
3.17624638273335),.UNSPECIFIED.);
#6422=B_SPLINE_CURVE_WITH_KNOTS('',3,(#272329,#272330,#272331,#272332,#272333,
#272334,#272335,#272336),.UNSPECIFIED.,.F.,.F.,(4,2,2,4),(-8.98049293428025,
-8.97889171867629,-8.34884827602915,-8.12983481856118),.UNSPECIFIED.);
#6423=B_SPLINE_CURVE_WITH_KNOTS('',3,(#272344,#272345,#272346,#272347),
 .UNSPECIFIED.,.F.,.F.,(4,4),(1.16920248436201,1.32846217039475),
 .UNSPECIFIED.);
#6424=B_SPLINE_CURVE_WITH_KNOTS('',3,(#272349,#272350,#272351,#272352,#272353,
#272354),.UNSPECIFIED.,.F.,.F.,(4,2,4),(-2.68771546706102,-2.29799156778106,
-1.97285776109958),.UNSPECIFIED.);
#6425=B_SPLINE_CURVE_WITH_KNOTS('',3,(#272356,#272357,#272358,#272359,#272360,
#272361),.UNSPECIFIED.,.F.,.F.,(4,2,4),(2.36444145675474,2.40335316041175,
2.5234386581235),.UNSPECIFIED.);
#7226=SHAPE_REPRESENTATION_RELATIONSHIP('SRR','None',#310899,#7243);
#7243=ADVANCED_BREP_SHAPE_REPRESENTATION('',(#7347,#7348),#310608);
#7279=STYLED_ITEM('',(#311003),#7347);
#7280=STYLED_ITEM('',(#311003),#7348);
#7347=MANIFOLD_SOLID_BREP('Body1',#93729);
#7348=MANIFOLD_SOLID_BREP('Body2',#93730);
#7622=FACE_BOUND('',#19617,.T.);
#7623=FACE_BOUND('',#19619,.T.);
#7624=FACE_BOUND('',#19666,.T.);
#7625=FACE_BOUND('',#19713,.T.);
#7626=FACE_BOUND('',#19715,.T.);
#8524=PLANE('',#103370);
#8525=PLANE('',#103395);
#8526=PLANE('',#103486);
#8527=PLANE('',#103533);
#8528=PLANE('',#103534);
#8529=PLANE('',#103535);
#8530=PLANE('',#103542);
#8531=PLANE('',#103543);
#8532=PLANE('',#103544);
#8533=PLANE('',#103545);
#8534=PLANE('',#103546);
#13635=FACE_OUTER_BOUND('',#19605,.T.);
#13636=FACE_OUTER_BOUND('',#19606,.T.);
#13637=FACE_OUTER_BOUND('',#19607,.T.);
#13638=FACE_OUTER_BOUND('',#19608,.T.);
#13639=FACE_OUTER_BOUND('',#19609,.T.);
#13640=FACE_OUTER_BOUND('',#19610,.T.);
#13641=FACE_OUTER_BOUND('',#19611,.T.);
#13642=FACE_OUTER_BOUND('',#19612,.T.);
#13643=FACE_OUTER_BOUND('',#19613,.T.);
#13644=FACE_OUTER_BOUND('',#19614,.T.);
#13645=FACE_OUTER_BOUND('',#19615,.T.);
#13646=FACE_OUTER_BOUND('',#19616,.T.);
#13647=FACE_OUTER_BOUND('',#19618,.T.);
#13648=FACE_OUTER_BOUND('',#19620,.T.);
#13649=FACE_OUTER_BOUND('',#19621,.T.);
#13650=FACE_OUTER_BOUND('',#19622,.T.);
#13651=FACE_OUTER_BOUND('',#19623,.T.);
#13652=FACE_OUTER_BOUND('',#19624,.T.);
#13653=FACE_OUTER_BOUND('',#19625,.T.);
#13654=FACE_OUTER_BOUND('',#19626,.T.);
#13655=FACE_OUTER_BOUND('',#19627,.T.);
#13656=FACE_OUTER_BOUND('',#19628,.T.);
#13657=FACE_OUTER_BOUND('',#19629,.T.);
#13658=FACE_OUTER_BOUND('',#19630,.T.);
#13659=FACE_OUTER_BOUND('',#19631,.T.);
#13660=FACE_OUTER_BOUND('',#19632,.T.);
#13661=FACE_OUTER_BOUND('',#19633,.T.);
#13662=FACE_OUTER_BOUND('',#19634,.T.);
#13663=FACE_OUTER_BOUND('',#19635,.T.);
#13664=FACE_OUTER_BOUND('',#19636,.T.);
#13665=FACE_OUTER_BOUND('',#19637,.T.);
#13666=FACE_OUTER_BOUND('',#19638,.T.);
#13667=FACE_OUTER_BOUND('',#19639,.T.);
#13668=FACE_OUTER_BOUND('',#19640,.T.);
#13669=FACE_OUTER_BOUND('',#19641,.T.);
#13670=FACE_OUTER_BOUND('',#19642,.T.);
#13671=FACE_OUTER_BOUND('',#19643,.T.);
#13672=FACE_OUTER_BOUND('',#19644,.T.);
#13673=FACE_OUTER_BOUND('',#19645,.T.);
#13674=FACE_OUTER_BOUND('',#19646,.T.);
#13675=FACE_OUTER_BOUND('',#19647,.T.);
#13676=FACE_OUTER_BOUND('',#19648,.T.);
#13677=FACE_OUTER_BOUND('',#19649,.T.);
#13678=FACE_OUTER_BOUND('',#19650,.T.);
#13679=FACE_OUTER_BOUND('',#19651,.T.);
#13680=FACE_OUTER_BOUND('',#19652,.T.);
#13681=FACE_OUTER_BOUND('',#19653,.T.);
#13682=FACE_OUTER_BOUND('',#19654,.T.);
#13683=FACE_OUTER_BOUND('',#19655,.T.);
#13684=FACE_OUTER_BOUND('',#19656,.T.);
#13685=FACE_OUTER_BOUND('',#19657,.T.);
#13686=FACE_OUTER_BOUND('',#19658,.T.);
#13687=FACE_OUTER_BOUND('',#19659,.T.);
#13688=FACE_OUTER_BOUND('',#19660,.T.);
#13689=FACE_OUTER_BOUND('',#19661,.T.);
#13690=FACE_OUTER_BOUND('',#19662,.T.);
#13691=FACE_OUTER_BOUND('',#19663,.T.);
#13692=FACE_OUTER_BOUND('',#19664,.T.);
#13693=FACE_OUTER_BOUND('',#19665,.T.);
#13694=FACE_OUTER_BOUND('',#19667,.T.);
#13695=FACE_OUTER_BOUND('',#19668,.T.);
#13696=FACE_OUTER_BOUND('',#19669,.T.);
#13697=FACE_OUTER_BOUND('',#19670,.T.);
#13698=FACE_OUTER_BOUND('',#19671,.T.);
#13699=FACE_OUTER_BOUND('',#19672,.T.);
#13700=FACE_OUTER_BOUND('',#19673,.T.);
#13701=FACE_OUTER_BOUND('',#19674,.T.);
#13702=FACE_OUTER_BOUND('',#19675,.T.);
#13703=FACE_OUTER_BOUND('',#19676,.T.);
#13704=FACE_OUTER_BOUND('',#19677,.T.);
#13705=FACE_OUTER_BOUND('',#19678,.T.);
#13706=FACE_OUTER_BOUND('',#19679,.T.);
#13707=FACE_OUTER_BOUND('',#19680,.T.);
#13708=FACE_OUTER_BOUND('',#19681,.T.);
#13709=FACE_OUTER_BOUND('',#19682,.T.);
#13710=FACE_OUTER_BOUND('',#19683,.T.);
#13711=FACE_OUTER_BOUND('',#19684,.T.);
#13712=FACE_OUTER_BOUND('',#19685,.T.);
#13713=FACE_OUTER_BOUND('',#19686,.T.);
#13714=FACE_OUTER_BOUND('',#19687,.T.);
#13715=FACE_OUTER_BOUND('',#19688,.T.);
#13716=FACE_OUTER_BOUND('',#19689,.T.);
#13717=FACE_OUTER_BOUND('',#19690,.T.);
#13718=FACE_OUTER_BOUND('',#19691,.T.);
#13719=FACE_OUTER_BOUND('',#19692,.T.);
#13720=FACE_OUTER_BOUND('',#19693,.T.);
#13721=FACE_OUTER_BOUND('',#19694,.T.);
#13722=FACE_OUTER_BOUND('',#19695,.T.);
#13723=FACE_OUTER_BOUND('',#19696,.T.);
#13724=FACE_OUTER_BOUND('',#19697,.T.);
#13725=FACE_OUTER_BOUND('',#19698,.T.);
#13726=FACE_OUTER_BOUND('',#19699,.T.);
#13727=FACE_OUTER_BOUND('',#19700,.T.);
#13728=FACE_OUTER_BOUND('',#19701,.T.);
#13729=FACE_OUTER_BOUND('',#19702,.T.);
#13730=FACE_OUTER_BOUND('',#19703,.T.);
#13731=FACE_OUTER_BOUND('',#19704,.T.);
#13732=FACE_OUTER_BOUND('',#19705,.T.);
#13733=FACE_OUTER_BOUND('',#19706,.T.);
#13734=FACE_OUTER_BOUND('',#19707,.T.);
#13735=FACE_OUTER_BOUND('',#19708,.T.);
#13736=FACE_OUTER_BOUND('',#19709,.T.);
#13737=FACE_OUTER_BOUND('',#19710,.T.);
#13738=FACE_OUTER_BOUND('',#19711,.T.);
#13739=FACE_OUTER_BOUND('',#19712,.T.);
#13740=FACE_OUTER_BOUND('',#19714,.T.);
#19605=EDGE_LOOP('',(#81717,#81718,#81719,#81720));
#19606=EDGE_LOOP('',(#81721,#81722,#81723,#81724));
#19607=EDGE_LOOP('',(#81725,#81726,#81727,#81728));
#19608=EDGE_LOOP('',(#81729,#81730,#81731,#81732,#81733,#81734,#81735,#81736));
#19609=EDGE_LOOP('',(#81737,#81738,#81739,#81740,#81741,#81742,#81743,#81744));
#19610=EDGE_LOOP('',(#81745,#81746,#81747,#81748,#81749,#81750,#81751,#81752));
#19611=EDGE_LOOP('',(#81753,#81754,#81755,#81756,#81757,#81758,#81759,#81760));
#19612=EDGE_LOOP('',(#81761,#81762,#81763,#81764,#81765,#81766,#81767,#81768));
#19613=EDGE_LOOP('',(#81769,#81770,#81771,#81772,#81773,#81774,#81775,#81776));
#19614=EDGE_LOOP('',(#81777,#81778,#81779,#81780));
#19615=EDGE_LOOP('',(#81781,#81782,#81783,#81784));
#19616=EDGE_LOOP('',(#81785,#81786,#81787,#81788,#81789,#81790,#81791,#81792,
#81793,#81794,#81795,#81796,#81797,#81798,#81799,#81800,#81801,#81802,#81803,
#81804,#81805,#81806,#81807,#81808,#81809,#81810,#81811,#81812,#81813,#81814));
#19617=EDGE_LOOP('',(#81815,#81816,#81817,#81818));
#19618=EDGE_LOOP('',(#81819));
#19619=EDGE_LOOP('',(#81820,#81821,#81822,#81823));
#19620=EDGE_LOOP('',(#81824,#81825,#81826,#81827,#81828,#81829));
#19621=EDGE_LOOP('',(#81830,#81831,#81832,#81833,#81834,#81835));
#19622=EDGE_LOOP('',(#81836,#81837,#81838,#81839,#81840,#81841));
#19623=EDGE_LOOP('',(#81842,#81843,#81844,#81845,#81846,#81847));
#19624=EDGE_LOOP('',(#81848,#81849,#81850,#81851,#81852,#81853));
#19625=EDGE_LOOP('',(#81854,#81855,#81856,#81857,#81858,#81859));
#19626=EDGE_LOOP('',(#81860,#81861,#81862,#81863,#81864,#81865));
#19627=EDGE_LOOP('',(#81866,#81867,#81868,#81869,#81870,#81871));
#19628=EDGE_LOOP('',(#81872,#81873,#81874,#81875,#81876,#81877));
#19629=EDGE_LOOP('',(#81878,#81879,#81880,#81881,#81882,#81883));
#19630=EDGE_LOOP('',(#81884,#81885,#81886,#81887,#81888,#81889));
#19631=EDGE_LOOP('',(#81890,#81891,#81892,#81893,#81894,#81895));
#19632=EDGE_LOOP('',(#81896,#81897,#81898,#81899,#81900,#81901));
#19633=EDGE_LOOP('',(#81902,#81903,#81904,#81905,#81906,#81907));
#19634=EDGE_LOOP('',(#81908,#81909,#81910,#81911));
#19635=EDGE_LOOP('',(#81912,#81913,#81914,#81915));
#19636=EDGE_LOOP('',(#81916,#81917,#81918,#81919));
#19637=EDGE_LOOP('',(#81920,#81921,#81922,#81923));
#19638=EDGE_LOOP('',(#81924,#81925,#81926,#81927));
#19639=EDGE_LOOP('',(#81928,#81929,#81930,#81931));
#19640=EDGE_LOOP('',(#81932,#81933,#81934,#81935));
#19641=EDGE_LOOP('',(#81936,#81937,#81938,#81939));
#19642=EDGE_LOOP('',(#81940,#81941,#81942,#81943));
#19643=EDGE_LOOP('',(#81944,#81945,#81946,#81947));
#19644=EDGE_LOOP('',(#81948,#81949,#81950,#81951));
#19645=EDGE_LOOP('',(#81952,#81953,#81954,#81955));
#19646=EDGE_LOOP('',(#81956,#81957,#81958,#81959));
#19647=EDGE_LOOP('',(#81960,#81961,#81962,#81963));
#19648=EDGE_LOOP('',(#81964,#81965,#81966,#81967,#81968,#81969));
#19649=EDGE_LOOP('',(#81970,#81971,#81972,#81973,#81974,#81975));
#19650=EDGE_LOOP('',(#81976,#81977,#81978,#81979,#81980,#81981));
#19651=EDGE_LOOP('',(#81982,#81983,#81984,#81985,#81986,#81987));
#19652=EDGE_LOOP('',(#81988,#81989,#81990,#81991,#81992,#81993));
#19653=EDGE_LOOP('',(#81994,#81995,#81996,#81997,#81998,#81999));
#19654=EDGE_LOOP('',(#82000,#82001,#82002,#82003,#82004,#82005));
#19655=EDGE_LOOP('',(#82006,#82007,#82008,#82009,#82010,#82011));
#19656=EDGE_LOOP('',(#82012,#82013,#82014,#82015,#82016,#82017));
#19657=EDGE_LOOP('',(#82018,#82019,#82020,#82021,#82022,#82023));
#19658=EDGE_LOOP('',(#82024,#82025,#82026,#82027,#82028,#82029));
#19659=EDGE_LOOP('',(#82030,#82031,#82032,#82033,#82034,#82035));
#19660=EDGE_LOOP('',(#82036,#82037,#82038,#82039,#82040,#82041));
#19661=EDGE_LOOP('',(#82042,#82043,#82044,#82045,#82046,#82047));
#19662=EDGE_LOOP('',(#82048,#82049,#82050,#82051,#82052,#82053));
#19663=EDGE_LOOP('',(#82054,#82055,#82056,#82057));
#19664=EDGE_LOOP('',(#82058,#82059,#82060,#82061,#82062,#82063));
#19665=EDGE_LOOP('',(#82064,#82065,#82066,#82067,#82068,#82069,#82070,#82071,
#82072,#82073,#82074,#82075,#82076,#82077,#82078,#82079,#82080,#82081,#82082,
#82083,#82084,#82085,#82086,#82087,#82088,#82089,#82090,#82091,#82092,#82093));
#19666=EDGE_LOOP('',(#82094));
#19667=EDGE_LOOP('',(#82095,#82096,#82097,#82098));
#19668=EDGE_LOOP('',(#82099,#82100,#82101,#82102));
#19669=EDGE_LOOP('',(#82103,#82104,#82105,#82106,#82107,#82108,#82109,#82110));
#19670=EDGE_LOOP('',(#82111,#82112,#82113,#82114));
#19671=EDGE_LOOP('',(#82115,#82116,#82117,#82118,#82119,#82120,#82121,#82122));
#19672=EDGE_LOOP('',(#82123,#82124,#82125,#82126));
#19673=EDGE_LOOP('',(#82127,#82128,#82129,#82130));
#19674=EDGE_LOOP('',(#82131,#82132,#82133,#82134));
#19675=EDGE_LOOP('',(#82135,#82136,#82137,#82138));
#19676=EDGE_LOOP('',(#82139,#82140,#82141,#82142));
#19677=EDGE_LOOP('',(#82143,#82144,#82145,#82146));
#19678=EDGE_LOOP('',(#82147,#82148,#82149,#82150));
#19679=EDGE_LOOP('',(#82151,#82152,#82153,#82154));
#19680=EDGE_LOOP('',(#82155,#82156,#82157,#82158));
#19681=EDGE_LOOP('',(#82159,#82160,#82161,#82162));
#19682=EDGE_LOOP('',(#82163,#82164,#82165,#82166,#82167,#82168,#82169,#82170));
#19683=EDGE_LOOP('',(#82171,#82172,#82173,#82174));
#19684=EDGE_LOOP('',(#82175,#82176,#82177,#82178));
#19685=EDGE_LOOP('',(#82179,#82180,#82181,#82182));
#19686=EDGE_LOOP('',(#82183,#82184,#82185,#82186));
#19687=EDGE_LOOP('',(#82187,#82188,#82189,#82190));
#19688=EDGE_LOOP('',(#82191,#82192,#82193,#82194));
#19689=EDGE_LOOP('',(#82195,#82196,#82197,#82198,#82199,#82200,#82201,#82202));
#19690=EDGE_LOOP('',(#82203,#82204,#82205,#82206));
#19691=EDGE_LOOP('',(#82207,#82208,#82209,#82210));
#19692=EDGE_LOOP('',(#82211,#82212,#82213,#82214,#82215,#82216,#82217,#82218));
#19693=EDGE_LOOP('',(#82219,#82220,#82221,#82222));
#19694=EDGE_LOOP('',(#82223,#82224,#82225,#82226,#82227,#82228,#82229,#82230));
#19695=EDGE_LOOP('',(#82231,#82232,#82233,#82234));
#19696=EDGE_LOOP('',(#82235,#82236,#82237,#82238));
#19697=EDGE_LOOP('',(#82239,#82240,#82241,#82242,#82243,#82244,#82245,#82246));
#19698=EDGE_LOOP('',(#82247,#82248,#82249,#82250));
#19699=EDGE_LOOP('',(#82251,#82252,#82253,#82254));
#19700=EDGE_LOOP('',(#82255,#82256,#82257,#82258,#82259,#82260,#82261,#82262));
#19701=EDGE_LOOP('',(#82263,#82264,#82265,#82266));
#19702=EDGE_LOOP('',(#82267,#82268,#82269,#82270));
#19703=EDGE_LOOP('',(#82271,#82272,#82273,#82274,#82275,#82276,#82277,#82278));
#19704=EDGE_LOOP('',(#82279,#82280,#82281,#82282));
#19705=EDGE_LOOP('',(#82283,#82284,#82285,#82286));
#19706=EDGE_LOOP('',(#82287,#82288,#82289,#82290));
#19707=EDGE_LOOP('',(#82291,#82292,#82293,#82294));
#19708=EDGE_LOOP('',(#82295,#82296,#82297,#82298));
#19709=EDGE_LOOP('',(#82299,#82300,#82301,#82302));
#19710=EDGE_LOOP('',(#82303,#82304,#82305,#82306));
#19711=EDGE_LOOP('',(#82307,#82308,#82309,#82310));
#19712=EDGE_LOOP('',(#82311,#82312,#82313,#82314));
#19713=EDGE_LOOP('',(#82315));
#19714=EDGE_LOOP('',(#82316,#82317,#82318,#82319));
#19715=EDGE_LOOP('',(#82320));
#24204=LINE('',#271232,#28551);
#24205=LINE('',#271246,#28552);
#24206=LINE('',#271254,#28553);
#24207=LINE('',#271265,#28554);
#24208=LINE('',#271281,#28555);
#24209=LINE('',#271302,#28556);
#24210=LINE('',#271318,#28557);
#24211=LINE('',#271337,#28558);
#24212=LINE('',#271353,#28559);
#24213=LINE('',#271379,#28560);
#24214=LINE('',#271394,#28561);
#24215=LINE('',#271407,#28562);
#24216=LINE('',#271423,#28563);
#24217=LINE('',#271442,#28564);
#24218=LINE('',#271458,#28565);
#24219=LINE('',#271475,#28566);
#24220=LINE('',#271485,#28567);
#24221=LINE('',#271491,#28568);
#24222=LINE('',#271494,#28569);
#24223=LINE('',#271539,#28570);
#24224=LINE('',#271541,#28571);
#24225=LINE('',#271542,#28572);
#24226=LINE('',#271545,#28573);
#24227=LINE('',#271547,#28574);
#24228=LINE('',#271548,#28575);
#24229=LINE('',#271905,#28576);
#24230=LINE('',#271908,#28577);
#24231=LINE('',#271911,#28578);
#24232=LINE('',#271913,#28579);
#24233=LINE('',#271917,#28580);
#24234=LINE('',#271919,#28581);
#24235=LINE('',#271923,#28582);
#24236=LINE('',#271925,#28583);
#24237=LINE('',#271930,#28584);
#24238=LINE('',#271933,#28585);
#24239=LINE('',#271935,#28586);
#24240=LINE('',#271939,#28587);
#24241=LINE('',#271942,#28588);
#24242=LINE('',#271945,#28589);
#24243=LINE('',#271948,#28590);
#24244=LINE('',#271951,#28591);
#24245=LINE('',#271953,#28592);
#24246=LINE('',#271957,#28593);
#24247=LINE('',#271960,#28594);
#24248=LINE('',#271963,#28595);
#24249=LINE('',#271966,#28596);
#24250=LINE('',#271969,#28597);
#24251=LINE('',#271971,#28598);
#24252=LINE('',#271975,#28599);
#24253=LINE('',#271978,#28600);
#24254=LINE('',#271981,#28601);
#24255=LINE('',#271983,#28602);
#24256=LINE('',#272340,#28603);
#24257=LINE('',#272374,#28604);
#24258=LINE('',#272376,#28605);
#24259=LINE('',#272379,#28606);
#24260=LINE('',#272390,#28607);
#24261=LINE('',#272392,#28608);
#24262=LINE('',#272399,#28609);
#24263=LINE('',#272401,#28610);
#24264=LINE('',#272404,#28611);
#24265=LINE('',#272406,#28612);
#24266=LINE('',#272409,#28613);
#24267=LINE('',#272412,#28614);
#24268=LINE('',#272414,#28615);
#24269=LINE('',#272417,#28616);
#24270=LINE('',#272419,#28617);
#24271=LINE('',#272422,#28618);
#24272=LINE('',#272424,#28619);
#24273=LINE('',#272427,#28620);
#24274=LINE('',#272428,#28621);
#24275=LINE('',#272435,#28622);
#24276=LINE('',#272442,#28623);
#24277=LINE('',#272445,#28624);
#24278=LINE('',#272448,#28625);
#24279=LINE('',#272450,#28626);
#24280=LINE('',#272451,#28627);
#24281=LINE('',#272454,#28628);
#24282=LINE('',#272456,#28629);
#24283=LINE('',#272457,#28630);
#24284=LINE('',#272459,#28631);
#24285=LINE('',#272460,#28632);
#28551=VECTOR('',#127353,32.4);
#28552=VECTOR('',#127358,1000.);
#28553=VECTOR('',#127359,1000.);
#28554=VECTOR('',#127362,1000.);
#28555=VECTOR('',#127365,1000.);
#28556=VECTOR('',#127372,1000.);
#28557=VECTOR('',#127375,1000.);
#28558=VECTOR('',#127380,1000.);
#28559=VECTOR('',#127383,1000.);
#28560=VECTOR('',#127388,1000.);
#28561=VECTOR('',#127391,1000.);
#28562=VECTOR('',#127396,1000.);
#28563=VECTOR('',#127399,1000.);
#28564=VECTOR('',#127404,1000.);
#28565=VECTOR('',#127407,1000.);
#28566=VECTOR('',#127410,1000.);
#28567=VECTOR('',#127411,1000.);
#28568=VECTOR('',#127416,1000.);
#28569=VECTOR('',#127419,1000.);
#28570=VECTOR('',#127470,1000.);
#28571=VECTOR('',#127471,1000.);
#28572=VECTOR('',#127472,1000.);
#28573=VECTOR('',#127475,1000.);
#28574=VECTOR('',#127476,1000.);
#28575=VECTOR('',#127477,1000.);
#28576=VECTOR('',#127536,1000.);
#28577=VECTOR('',#127539,1000.);
#28578=VECTOR('',#127542,1000.);
#28579=VECTOR('',#127543,1000.);
#28580=VECTOR('',#127548,1000.);
#28581=VECTOR('',#127549,1000.);
#28582=VECTOR('',#127554,1000.);
#28583=VECTOR('',#127555,1000.);
#28584=VECTOR('',#127562,1000.);
#28585=VECTOR('',#127565,1000.);
#28586=VECTOR('',#127566,1000.);
#28587=VECTOR('',#127571,1000.);
#28588=VECTOR('',#127574,1000.);
#28589=VECTOR('',#127577,1000.);
#28590=VECTOR('',#127580,1000.);
#28591=VECTOR('',#127583,1000.);
#28592=VECTOR('',#127584,1000.);
#28593=VECTOR('',#127589,1000.);
#28594=VECTOR('',#127592,1000.);
#28595=VECTOR('',#127595,1000.);
#28596=VECTOR('',#127598,1000.);
#28597=VECTOR('',#127601,1000.);
#28598=VECTOR('',#127602,1000.);
#28599=VECTOR('',#127607,1000.);
#28600=VECTOR('',#127610,1000.);
#28601=VECTOR('',#127613,1000.);
#28602=VECTOR('',#127614,1000.);
#28603=VECTOR('',#127679,1000.);
#28604=VECTOR('',#127708,1000.);
#28605=VECTOR('',#127711,1000.);
#28606=VECTOR('',#127716,1000.);
#28607=VECTOR('',#127737,1000.);
#28608=VECTOR('',#127740,1000.);
#28609=VECTOR('',#127753,1000.);
#28610=VECTOR('',#127756,1000.);
#28611=VECTOR('',#127761,1000.);
#28612=VECTOR('',#127764,1000.);
#28613=VECTOR('',#127769,1000.);
#28614=VECTOR('',#127774,1000.);
#28615=VECTOR('',#127777,1000.);
#28616=VECTOR('',#127782,1000.);
#28617=VECTOR('',#127785,1000.);
#28618=VECTOR('',#127790,1000.);
#28619=VECTOR('',#127793,1000.);
#28620=VECTOR('',#127798,1000.);
#28621=VECTOR('',#127799,1000.);
#28622=VECTOR('',#127808,10.12);
#28623=VECTOR('',#127815,1000.);
#28624=VECTOR('',#127818,1000.);
#28625=VECTOR('',#127821,1000.);
#28626=VECTOR('',#127822,1000.);
#28627=VECTOR('',#127823,1000.);
#28628=VECTOR('',#127826,1000.);
#28629=VECTOR('',#127827,1000.);
#28630=VECTOR('',#127828,1000.);
#28631=VECTOR('',#127831,1000.);
#28632=VECTOR('',#127832,1000.);
#34565=CIRCLE('',#103342,32.976);
#34566=CIRCLE('',#103343,0.576);
#34567=CIRCLE('',#103344,32.4);
#34568=CIRCLE('',#103346,32.4);
#34569=CIRCLE('',#103349,5.77396800000001);
#34570=CIRCLE('',#103350,5.77396800000001);
#34571=CIRCLE('',#103352,5.773968);
#34572=CIRCLE('',#103353,5.77396800000001);
#34573=CIRCLE('',#103355,5.773968);
#34574=CIRCLE('',#103356,5.773968);
#34575=CIRCLE('',#103358,5.773968);
#34576=CIRCLE('',#103359,5.77396800000001);
#34577=CIRCLE('',#103361,5.773968);
#34578=CIRCLE('',#103362,5.77396800000001);
#34579=CIRCLE('',#103364,5.77396800000001);
#34580=CIRCLE('',#103365,5.77396800000001);
#34581=CIRCLE('',#103368,15.12);
#34582=CIRCLE('',#103369,15.12);
#34583=CIRCLE('',#103371,5.77396800000001);
#34584=CIRCLE('',#103372,40.6764810164406);
#34585=CIRCLE('',#103373,5.773968);
#34586=CIRCLE('',#103374,40.6764810164406);
#34587=CIRCLE('',#103375,5.773968);
#34588=CIRCLE('',#103376,40.6764810164406);
#34589=CIRCLE('',#103377,5.773968);
#34590=CIRCLE('',#103378,40.6764810164406);
#34591=CIRCLE('',#103379,5.77396800000001);
#34592=CIRCLE('',#103380,40.6764810164406);
#34593=CIRCLE('',#103381,40.6764810164406);
#34594=CIRCLE('',#103382,40.6764810164406);
#34595=CIRCLE('',#103383,40.6764810164406);
#34596=CIRCLE('',#103384,40.6764810164406);
#34597=CIRCLE('',#103385,40.6764810164406);
#34598=CIRCLE('',#103386,40.6764810164406);
#34599=CIRCLE('',#103387,5.77396800000001);
#34600=CIRCLE('',#103388,40.6764810164406);
#34601=CIRCLE('',#103389,5.773968);
#34602=CIRCLE('',#103390,40.6764810164406);
#34603=CIRCLE('',#103391,5.77396800000001);
#34604=CIRCLE('',#103392,40.6764810164406);
#34605=CIRCLE('',#103393,5.773968);
#34606=CIRCLE('',#103394,40.6764810164406);
#34607=CIRCLE('',#103397,49.6934108978581);
#34608=CIRCLE('',#103399,49.6934108978581);
#34609=CIRCLE('',#103401,49.6934108978581);
#34610=CIRCLE('',#103403,49.6934108978581);
#34611=CIRCLE('',#103405,49.6934108978581);
#34612=CIRCLE('',#103407,49.6934108978581);
#34613=CIRCLE('',#103409,49.6934108978581);
#34614=CIRCLE('',#103411,49.6934108978581);
#34615=CIRCLE('',#103413,49.6934108978581);
#34616=CIRCLE('',#103415,49.6934108978581);
#34617=CIRCLE('',#103417,49.6934108978581);
#34618=CIRCLE('',#103419,49.6934108978581);
#34619=CIRCLE('',#103421,49.6934108978581);
#34620=CIRCLE('',#103423,49.6934108978581);
#34621=CIRCLE('',#103425,49.6934108978581);
#34622=CIRCLE('',#103427,49.6934108978581);
#34623=CIRCLE('',#103429,49.6934108978581);
#34624=CIRCLE('',#103431,49.6934108978581);
#34625=CIRCLE('',#103433,49.6934108978581);
#34626=CIRCLE('',#103435,49.6934108978581);
#34627=CIRCLE('',#103437,49.6934108978581);
#34628=CIRCLE('',#103439,49.6934108978581);
#34629=CIRCLE('',#103441,49.6934108978581);
#34630=CIRCLE('',#103443,49.6934108978581);
#34631=CIRCLE('',#103445,49.6934108978581);
#34632=CIRCLE('',#103447,49.6934108978581);
#34633=CIRCLE('',#103449,49.6934108978581);
#34634=CIRCLE('',#103451,49.6934108978581);
#34635=CIRCLE('',#103453,40.6764810164406);
#34636=CIRCLE('',#103455,40.6764810164406);
#34637=CIRCLE('',#103457,40.6764810164406);
#34638=CIRCLE('',#103459,40.6764810164406);
#34639=CIRCLE('',#103461,40.6764810164406);
#34640=CIRCLE('',#103463,40.6764810164406);
#34641=CIRCLE('',#103465,40.6764810164406);
#34642=CIRCLE('',#103467,40.6764810164406);
#34643=CIRCLE('',#103469,40.6764810164406);
#34644=CIRCLE('',#103471,40.6764810164406);
#34645=CIRCLE('',#103473,40.6764810164406);
#34646=CIRCLE('',#103475,40.6764810164406);
#34647=CIRCLE('',#103477,40.6764810164406);
#34648=CIRCLE('',#103479,40.6764810164406);
#34649=CIRCLE('',#103481,49.6934108978581);
#34650=CIRCLE('',#103483,49.6934108978581);
#34651=CIRCLE('',#103485,40.6764810164406);
#34652=CIRCLE('',#103487,5.77396800000001);
#34653=CIRCLE('',#103488,5.77396800000001);
#34654=CIRCLE('',#103489,5.77396800000001);
#34655=CIRCLE('',#103490,5.77396800000001);
#34656=CIRCLE('',#103491,5.773968);
#34657=CIRCLE('',#103492,5.77396800000001);
#34658=CIRCLE('',#103493,5.773968);
#34659=CIRCLE('',#103494,5.77396800000001);
#34660=CIRCLE('',#103495,5.77396800000001);
#34661=CIRCLE('',#103537,10.12);
#34662=CIRCLE('',#103538,10.12);
#34663=CIRCLE('',#103540,15.12);
#34664=CIRCLE('',#103541,15.12);
#42253=VERTEX_POINT('',#271225);
#42254=VERTEX_POINT('',#271227);
#42255=VERTEX_POINT('',#271231);
#42256=VERTEX_POINT('',#271235);
#42257=VERTEX_POINT('',#271236);
#42258=VERTEX_POINT('',#271245);
#42259=VERTEX_POINT('',#271247);
#42260=VERTEX_POINT('',#271256);
#42261=VERTEX_POINT('',#271257);
#42262=VERTEX_POINT('',#271264);
#42263=VERTEX_POINT('',#271266);
#42264=VERTEX_POINT('',#271271);
#42265=VERTEX_POINT('',#271273);
#42266=VERTEX_POINT('',#271280);
#42267=VERTEX_POINT('',#271282);
#42268=VERTEX_POINT('',#271291);
#42269=VERTEX_POINT('',#271292);
#42270=VERTEX_POINT('',#271294);
#42271=VERTEX_POINT('',#271301);
#42272=VERTEX_POINT('',#271303);
#42273=VERTEX_POINT('',#271308);
#42274=VERTEX_POINT('',#271310);
#42275=VERTEX_POINT('',#271317);
#42276=VERTEX_POINT('',#271326);
#42277=VERTEX_POINT('',#271327);
#42278=VERTEX_POINT('',#271329);
#42279=VERTEX_POINT('',#271336);
#42280=VERTEX_POINT('',#271338);
#42281=VERTEX_POINT('',#271343);
#42282=VERTEX_POINT('',#271345);
#42283=VERTEX_POINT('',#271352);
#42284=VERTEX_POINT('',#271361);
#42285=VERTEX_POINT('',#271362);
#42286=VERTEX_POINT('',#271369);
#42287=VERTEX_POINT('',#271371);
#42288=VERTEX_POINT('',#271378);
#42289=VERTEX_POINT('',#271380);
#42290=VERTEX_POINT('',#271385);
#42291=VERTEX_POINT('',#271387);
#42292=VERTEX_POINT('',#271396);
#42293=VERTEX_POINT('',#271397);
#42294=VERTEX_POINT('',#271399);
#42295=VERTEX_POINT('',#271406);
#42296=VERTEX_POINT('',#271408);
#42297=VERTEX_POINT('',#271413);
#42298=VERTEX_POINT('',#271415);
#42299=VERTEX_POINT('',#271422);
#42300=VERTEX_POINT('',#271431);
#42301=VERTEX_POINT('',#271432);
#42302=VERTEX_POINT('',#271434);
#42303=VERTEX_POINT('',#271441);
#42304=VERTEX_POINT('',#271443);
#42305=VERTEX_POINT('',#271448);
#42306=VERTEX_POINT('',#271450);
#42307=VERTEX_POINT('',#271457);
#42308=VERTEX_POINT('',#271466);
#42309=VERTEX_POINT('',#271467);
#42310=VERTEX_POINT('',#271474);
#42311=VERTEX_POINT('',#271476);
#42312=VERTEX_POINT('',#271487);
#42313=VERTEX_POINT('',#271488);
#42314=VERTEX_POINT('',#271490);
#42315=VERTEX_POINT('',#271492);
#42316=VERTEX_POINT('',#271496);
#42317=VERTEX_POINT('',#271497);
#42318=VERTEX_POINT('',#271499);
#42319=VERTEX_POINT('',#271501);
#42320=VERTEX_POINT('',#271503);
#42321=VERTEX_POINT('',#271505);
#42322=VERTEX_POINT('',#271507);
#42323=VERTEX_POINT('',#271509);
#42324=VERTEX_POINT('',#271511);
#42325=VERTEX_POINT('',#271513);
#42326=VERTEX_POINT('',#271521);
#42327=VERTEX_POINT('',#271523);
#42328=VERTEX_POINT('',#271525);
#42329=VERTEX_POINT('',#271527);
#42330=VERTEX_POINT('',#271529);
#42331=VERTEX_POINT('',#271531);
#42332=VERTEX_POINT('',#271533);
#42333=VERTEX_POINT('',#271535);
#42334=VERTEX_POINT('',#271538);
#42335=VERTEX_POINT('',#271540);
#42336=VERTEX_POINT('',#271544);
#42337=VERTEX_POINT('',#271546);
#42338=VERTEX_POINT('',#271550);
#42339=VERTEX_POINT('',#271551);
#42340=VERTEX_POINT('',#271560);
#42341=VERTEX_POINT('',#271562);
#42342=VERTEX_POINT('',#271582);
#42343=VERTEX_POINT('',#271589);
#42344=VERTEX_POINT('',#271596);
#42345=VERTEX_POINT('',#271605);
#42346=VERTEX_POINT('',#271614);
#42347=VERTEX_POINT('',#271621);
#42348=VERTEX_POINT('',#271628);
#42349=VERTEX_POINT('',#271637);
#42350=VERTEX_POINT('',#271646);
#42351=VERTEX_POINT('',#271653);
#42352=VERTEX_POINT('',#271660);
#42353=VERTEX_POINT('',#271669);
#42354=VERTEX_POINT('',#271678);
#42355=VERTEX_POINT('',#271680);
#42356=VERTEX_POINT('',#271700);
#42357=VERTEX_POINT('',#271707);
#42358=VERTEX_POINT('',#271714);
#42359=VERTEX_POINT('',#271723);
#42360=VERTEX_POINT('',#271732);
#42361=VERTEX_POINT('',#271733);
#42362=VERTEX_POINT('',#271742);
#42363=VERTEX_POINT('',#271744);
#42364=VERTEX_POINT('',#271764);
#42365=VERTEX_POINT('',#271773);
#42366=VERTEX_POINT('',#271782);
#42367=VERTEX_POINT('',#271789);
#42368=VERTEX_POINT('',#271798);
#42369=VERTEX_POINT('',#271807);
#42370=VERTEX_POINT('',#271816);
#42371=VERTEX_POINT('',#271825);
#42372=VERTEX_POINT('',#271834);
#42373=VERTEX_POINT('',#271843);
#42374=VERTEX_POINT('',#271852);
#42375=VERTEX_POINT('',#271861);
#42376=VERTEX_POINT('',#271870);
#42377=VERTEX_POINT('',#271872);
#42378=VERTEX_POINT('',#271886);
#42379=VERTEX_POINT('',#271895);
#42380=VERTEX_POINT('',#271904);
#42381=VERTEX_POINT('',#271906);
#42382=VERTEX_POINT('',#271910);
#42383=VERTEX_POINT('',#271912);
#42384=VERTEX_POINT('',#271916);
#42385=VERTEX_POINT('',#271918);
#42386=VERTEX_POINT('',#271922);
#42387=VERTEX_POINT('',#271924);
#42388=VERTEX_POINT('',#271928);
#42389=VERTEX_POINT('',#271932);
#42390=VERTEX_POINT('',#271934);
#42391=VERTEX_POINT('',#271938);
#42392=VERTEX_POINT('',#271940);
#42393=VERTEX_POINT('',#271944);
#42394=VERTEX_POINT('',#271946);
#42395=VERTEX_POINT('',#271950);
#42396=VERTEX_POINT('',#271952);
#42397=VERTEX_POINT('',#271956);
#42398=VERTEX_POINT('',#271958);
#42399=VERTEX_POINT('',#271962);
#42400=VERTEX_POINT('',#271964);
#42401=VERTEX_POINT('',#271968);
#42402=VERTEX_POINT('',#271970);
#42403=VERTEX_POINT('',#271974);
#42404=VERTEX_POINT('',#271976);
#42405=VERTEX_POINT('',#271980);
#42406=VERTEX_POINT('',#271982);
#42407=VERTEX_POINT('',#271986);
#42408=VERTEX_POINT('',#271993);
#42409=VERTEX_POINT('',#272000);
#42410=VERTEX_POINT('',#272002);
#42411=VERTEX_POINT('',#272016);
#42412=VERTEX_POINT('',#272017);
#42413=VERTEX_POINT('',#272030);
#42414=VERTEX_POINT('',#272037);
#42415=VERTEX_POINT('',#272046);
#42416=VERTEX_POINT('',#272047);
#42417=VERTEX_POINT('',#272060);
#42418=VERTEX_POINT('',#272067);
#42419=VERTEX_POINT('',#272076);
#42420=VERTEX_POINT('',#272077);
#42421=VERTEX_POINT('',#272090);
#42422=VERTEX_POINT('',#272097);
#42423=VERTEX_POINT('',#272106);
#42424=VERTEX_POINT('',#272113);
#42425=VERTEX_POINT('',#272115);
#42426=VERTEX_POINT('',#272129);
#42427=VERTEX_POINT('',#272130);
#42428=VERTEX_POINT('',#272143);
#42429=VERTEX_POINT('',#272150);
#42430=VERTEX_POINT('',#272159);
#42431=VERTEX_POINT('',#272166);
#42432=VERTEX_POINT('',#272173);
#42433=VERTEX_POINT('',#272175);
#42434=VERTEX_POINT('',#272213);
#42435=VERTEX_POINT('',#272220);
#42436=VERTEX_POINT('',#272283);
#42437=VERTEX_POINT('',#272285);
#42438=VERTEX_POINT('',#272321);
#42439=VERTEX_POINT('',#272328);
#42440=VERTEX_POINT('',#272339);
#42441=VERTEX_POINT('',#272343);
#42442=VERTEX_POINT('',#272348);
#42443=VERTEX_POINT('',#272355);
#42444=VERTEX_POINT('',#272432);
#42445=VERTEX_POINT('',#272434);
#42446=VERTEX_POINT('',#272438);
#42447=VERTEX_POINT('',#272439);
#42448=VERTEX_POINT('',#272441);
#42449=VERTEX_POINT('',#272443);
#42450=VERTEX_POINT('',#272447);
#42451=VERTEX_POINT('',#272449);
#42452=VERTEX_POINT('',#272453);
#42453=VERTEX_POINT('',#272455);
#55638=EDGE_CURVE('',#42253,#42253,#34565,.T.);
#55639=EDGE_CURVE('',#42253,#42254,#34566,.T.);
#55640=EDGE_CURVE('',#42254,#42254,#34567,.T.);
#55641=EDGE_CURVE('',#42254,#42255,#24204,.T.);
#55642=EDGE_CURVE('',#42255,#42255,#34568,.T.);
#55643=EDGE_CURVE('',#42256,#42257,#6306,.T.);
#55644=EDGE_CURVE('',#42257,#42258,#24205,.T.);
#55645=EDGE_CURVE('',#42258,#42259,#6307,.T.);
#55646=EDGE_CURVE('',#42259,#42256,#24206,.T.);
#55647=EDGE_CURVE('',#42260,#42261,#6308,.T.);
#55648=EDGE_CURVE('',#42261,#42262,#24207,.T.);
#55649=EDGE_CURVE('',#42262,#42263,#6309,.T.);
#55650=EDGE_CURVE('',#42263,#42264,#34569,.T.);
#55651=EDGE_CURVE('',#42264,#42265,#6310,.T.);
#55652=EDGE_CURVE('',#42266,#42265,#24208,.T.);
#55653=EDGE_CURVE('',#42266,#42267,#6311,.T.);
#55654=EDGE_CURVE('',#42267,#42260,#34570,.T.);
#55655=EDGE_CURVE('',#42268,#42269,#34571,.T.);
#55656=EDGE_CURVE('',#42269,#42270,#6312,.T.);
#55657=EDGE_CURVE('',#42270,#42271,#24209,.T.);
#55658=EDGE_CURVE('',#42271,#42272,#6313,.T.);
#55659=EDGE_CURVE('',#42272,#42273,#34572,.T.);
#55660=EDGE_CURVE('',#42273,#42274,#6314,.T.);
#55661=EDGE_CURVE('',#42275,#42274,#24210,.T.);
#55662=EDGE_CURVE('',#42275,#42268,#6315,.T.);
#55663=EDGE_CURVE('',#42276,#42277,#34573,.T.);
#55664=EDGE_CURVE('',#42277,#42278,#6316,.T.);
#55665=EDGE_CURVE('',#42278,#42279,#24211,.T.);
#55666=EDGE_CURVE('',#42279,#42280,#6317,.T.);
#55667=EDGE_CURVE('',#42280,#42281,#34574,.T.);
#55668=EDGE_CURVE('',#42281,#42282,#6318,.T.);
#55669=EDGE_CURVE('',#42283,#42282,#24212,.T.);
#55670=EDGE_CURVE('',#42283,#42276,#6319,.T.);
#55671=EDGE_CURVE('',#42284,#42285,#6320,.T.);
#55672=EDGE_CURVE('',#42285,#42286,#34575,.T.);
#55673=EDGE_CURVE('',#42286,#42287,#6321,.T.);
#55674=EDGE_CURVE('',#42287,#42288,#24213,.T.);
#55675=EDGE_CURVE('',#42288,#42289,#6322,.T.);
#55676=EDGE_CURVE('',#42289,#42290,#34576,.T.);
#55677=EDGE_CURVE('',#42290,#42291,#6323,.T.);
#55678=EDGE_CURVE('',#42284,#42291,#24214,.T.);
#55679=EDGE_CURVE('',#42292,#42293,#34577,.T.);
#55680=EDGE_CURVE('',#42293,#42294,#6324,.T.);
#55681=EDGE_CURVE('',#42294,#42295,#24215,.T.);
#55682=EDGE_CURVE('',#42295,#42296,#6325,.T.);
#55683=EDGE_CURVE('',#42296,#42297,#34578,.T.);
#55684=EDGE_CURVE('',#42297,#42298,#6326,.T.);
#55685=EDGE_CURVE('',#42299,#42298,#24216,.T.);
#55686=EDGE_CURVE('',#42299,#42292,#6327,.T.);
#55687=EDGE_CURVE('',#42300,#42301,#34579,.T.);
#55688=EDGE_CURVE('',#42301,#42302,#6328,.T.);
#55689=EDGE_CURVE('',#42302,#42303,#24217,.T.);
#55690=EDGE_CURVE('',#42303,#42304,#6329,.T.);
#55691=EDGE_CURVE('',#42304,#42305,#34580,.T.);
#55692=EDGE_CURVE('',#42305,#42306,#6330,.T.);
#55693=EDGE_CURVE('',#42307,#42306,#24218,.T.);
#55694=EDGE_CURVE('',#42307,#42300,#6331,.T.);
#55695=EDGE_CURVE('',#42308,#42309,#6332,.T.);
#55696=EDGE_CURVE('',#42309,#42310,#24219,.T.);
#55697=EDGE_CURVE('',#42310,#42311,#6333,.T.);
#55698=EDGE_CURVE('',#42308,#42311,#24220,.T.);
#55699=EDGE_CURVE('',#42312,#42313,#34581,.T.);
#55700=EDGE_CURVE('',#42313,#42314,#24221,.T.);
#55701=EDGE_CURVE('',#42315,#42314,#34582,.T.);
#55702=EDGE_CURVE('',#42315,#42312,#24222,.T.);
#55703=EDGE_CURVE('',#42316,#42317,#34583,.T.);
#55704=EDGE_CURVE('',#42318,#42316,#34584,.T.);
#55705=EDGE_CURVE('',#42319,#42318,#34585,.T.);
#55706=EDGE_CURVE('',#42320,#42319,#34586,.T.);
#55707=EDGE_CURVE('',#42321,#42320,#34587,.T.);
#55708=EDGE_CURVE('',#42322,#42321,#34588,.T.);
#55709=EDGE_CURVE('',#42323,#42322,#34589,.T.);
#55710=EDGE_CURVE('',#42324,#42323,#34590,.T.);
#55711=EDGE_CURVE('',#42325,#42324,#34591,.T.);
#55712=EDGE_CURVE('',#42260,#42325,#34592,.T.);
#55713=EDGE_CURVE('',#42269,#42267,#34593,.T.);
#55714=EDGE_CURVE('',#42301,#42268,#34594,.T.);
#55715=EDGE_CURVE('',#42293,#42300,#34595,.T.);
#55716=EDGE_CURVE('',#42277,#42292,#34596,.T.);
#55717=EDGE_CURVE('',#42286,#42276,#34597,.T.);
#55718=EDGE_CURVE('',#42326,#42285,#34598,.T.);
#55719=EDGE_CURVE('',#42327,#42326,#34599,.T.);
#55720=EDGE_CURVE('',#42328,#42327,#34600,.T.);
#55721=EDGE_CURVE('',#42329,#42328,#34601,.T.);
#55722=EDGE_CURVE('',#42330,#42329,#34602,.T.);
#55723=EDGE_CURVE('',#42331,#42330,#34603,.T.);
#55724=EDGE_CURVE('',#42332,#42331,#34604,.T.);
#55725=EDGE_CURVE('',#42333,#42332,#34605,.T.);
#55726=EDGE_CURVE('',#42317,#42333,#34606,.T.);
#55727=EDGE_CURVE('',#42313,#42334,#24223,.T.);
#55728=EDGE_CURVE('',#42335,#42312,#24224,.T.);
#55729=EDGE_CURVE('',#42334,#42335,#24225,.T.);
#55730=EDGE_CURVE('',#42314,#42336,#24226,.T.);
#55731=EDGE_CURVE('',#42336,#42337,#24227,.T.);
#55732=EDGE_CURVE('',#42337,#42315,#24228,.T.);
#55733=EDGE_CURVE('',#42338,#42339,#6334,.T.);
#55734=EDGE_CURVE('',#42340,#42338,#34607,.T.);
#55735=EDGE_CURVE('',#42341,#42340,#6335,.T.);
#55736=EDGE_CURVE('',#42318,#42341,#6336,.T.);
#55737=EDGE_CURVE('',#42339,#42316,#6337,.T.);
#55738=EDGE_CURVE('',#42317,#42342,#6338,.T.);
#55739=EDGE_CURVE('',#42343,#42333,#6339,.T.);
#55740=EDGE_CURVE('',#42344,#42343,#6340,.T.);
#55741=EDGE_CURVE('',#42345,#42344,#34608,.T.);
#55742=EDGE_CURVE('',#42342,#42345,#6341,.T.);
#55743=EDGE_CURVE('',#42332,#42346,#6342,.T.);
#55744=EDGE_CURVE('',#42347,#42331,#6343,.T.);
#55745=EDGE_CURVE('',#42348,#42347,#6344,.T.);
#55746=EDGE_CURVE('',#42349,#42348,#34609,.T.);
#55747=EDGE_CURVE('',#42346,#42349,#6345,.T.);
#55748=EDGE_CURVE('',#42330,#42350,#6346,.T.);
#55749=EDGE_CURVE('',#42351,#42329,#6347,.T.);
#55750=EDGE_CURVE('',#42352,#42351,#6348,.T.);
#55751=EDGE_CURVE('',#42353,#42352,#34610,.T.);
#55752=EDGE_CURVE('',#42350,#42353,#6349,.T.);
#55753=EDGE_CURVE('',#42354,#42256,#34611,.T.);
#55754=EDGE_CURVE('',#42355,#42354,#6350,.T.);
#55755=EDGE_CURVE('',#42322,#42355,#6351,.T.);
#55756=EDGE_CURVE('',#42257,#42321,#6352,.T.);
#55757=EDGE_CURVE('',#42320,#42356,#6353,.T.);
#55758=EDGE_CURVE('',#42357,#42319,#6354,.T.);
#55759=EDGE_CURVE('',#42358,#42357,#6355,.T.);
#55760=EDGE_CURVE('',#42359,#42358,#34612,.T.);
#55761=EDGE_CURVE('',#42356,#42359,#6356,.T.);
#55762=EDGE_CURVE('',#42360,#42361,#6357,.T.);
#55763=EDGE_CURVE('',#42362,#42360,#34613,.T.);
#55764=EDGE_CURVE('',#42363,#42362,#6358,.T.);
#55765=EDGE_CURVE('',#42324,#42363,#6359,.T.);
#55766=EDGE_CURVE('',#42361,#42323,#6360,.T.);
#55767=EDGE_CURVE('',#42364,#42266,#6361,.T.);
#55768=EDGE_CURVE('',#42365,#42364,#34614,.T.);
#55769=EDGE_CURVE('',#42270,#42365,#6362,.T.);
#55770=EDGE_CURVE('',#42366,#42325,#6363,.T.);
#55771=EDGE_CURVE('',#42367,#42366,#6364,.T.);
#55772=EDGE_CURVE('',#42368,#42367,#34615,.T.);
#55773=EDGE_CURVE('',#42261,#42368,#6365,.T.);
#55774=EDGE_CURVE('',#42369,#42275,#6366,.T.);
#55775=EDGE_CURVE('',#42370,#42369,#34616,.T.);
#55776=EDGE_CURVE('',#42302,#42370,#6367,.T.);
#55777=EDGE_CURVE('',#42371,#42283,#6368,.T.);
#55778=EDGE_CURVE('',#42372,#42371,#34617,.T.);
#55779=EDGE_CURVE('',#42287,#42372,#6369,.T.);
#55780=EDGE_CURVE('',#42373,#42299,#6370,.T.);
#55781=EDGE_CURVE('',#42374,#42373,#34618,.T.);
#55782=EDGE_CURVE('',#42278,#42374,#6371,.T.);
#55783=EDGE_CURVE('',#42375,#42284,#6372,.T.);
#55784=EDGE_CURVE('',#42376,#42375,#34619,.T.);
#55785=EDGE_CURVE('',#42377,#42376,#6373,.T.);
#55786=EDGE_CURVE('',#42326,#42377,#6374,.T.);
#55787=EDGE_CURVE('',#42378,#42307,#6375,.T.);
#55788=EDGE_CURVE('',#42379,#42378,#34620,.T.);
#55789=EDGE_CURVE('',#42294,#42379,#6376,.T.);
#55790=EDGE_CURVE('',#42380,#42338,#24229,.T.);
#55791=EDGE_CURVE('',#42381,#42380,#34621,.T.);
#55792=EDGE_CURVE('',#42340,#42381,#24230,.T.);
#55793=EDGE_CURVE('',#42345,#42382,#24231,.T.);
#55794=EDGE_CURVE('',#42383,#42344,#24232,.T.);
#55795=EDGE_CURVE('',#42382,#42383,#34622,.T.);
#55796=EDGE_CURVE('',#42349,#42384,#24233,.T.);
#55797=EDGE_CURVE('',#42385,#42348,#24234,.T.);
#55798=EDGE_CURVE('',#42384,#42385,#34623,.T.);
#55799=EDGE_CURVE('',#42353,#42386,#24235,.T.);
#55800=EDGE_CURVE('',#42387,#42352,#24236,.T.);
#55801=EDGE_CURVE('',#42386,#42387,#34624,.T.);
#55802=EDGE_CURVE('',#42388,#42259,#34625,.T.);
#55803=EDGE_CURVE('',#42354,#42388,#24237,.T.);
#55804=EDGE_CURVE('',#42359,#42389,#24238,.T.);
#55805=EDGE_CURVE('',#42390,#42358,#24239,.T.);
#55806=EDGE_CURVE('',#42389,#42390,#34626,.T.);
#55807=EDGE_CURVE('',#42391,#42360,#24240,.T.);
#55808=EDGE_CURVE('',#42392,#42391,#34627,.T.);
#55809=EDGE_CURVE('',#42362,#42392,#24241,.T.);
#55810=EDGE_CURVE('',#42393,#42364,#24242,.T.);
#55811=EDGE_CURVE('',#42394,#42393,#34628,.T.);
#55812=EDGE_CURVE('',#42365,#42394,#24243,.T.);
#55813=EDGE_CURVE('',#42368,#42395,#24244,.T.);
#55814=EDGE_CURVE('',#42396,#42367,#24245,.T.);
#55815=EDGE_CURVE('',#42395,#42396,#34629,.T.);
#55816=EDGE_CURVE('',#42397,#42369,#24246,.T.);
#55817=EDGE_CURVE('',#42398,#42397,#34630,.T.);
#55818=EDGE_CURVE('',#42370,#42398,#24247,.T.);
#55819=EDGE_CURVE('',#42399,#42371,#24248,.T.);
#55820=EDGE_CURVE('',#42400,#42399,#34631,.T.);
#55821=EDGE_CURVE('',#42372,#42400,#24249,.T.);
#55822=EDGE_CURVE('',#42374,#42401,#24250,.T.);
#55823=EDGE_CURVE('',#42402,#42373,#24251,.T.);
#55824=EDGE_CURVE('',#42401,#42402,#34632,.T.);
#55825=EDGE_CURVE('',#42403,#42375,#24252,.T.);
#55826=EDGE_CURVE('',#42404,#42403,#34633,.T.);
#55827=EDGE_CURVE('',#42376,#42404,#24253,.T.);
#55828=EDGE_CURVE('',#42379,#42405,#24254,.T.);
#55829=EDGE_CURVE('',#42406,#42378,#24255,.T.);
#55830=EDGE_CURVE('',#42405,#42406,#34634,.T.);
#55831=EDGE_CURVE('',#42407,#42380,#6377,.T.);
#55832=EDGE_CURVE('',#42408,#42407,#6378,.T.);
#55833=EDGE_CURVE('',#42409,#42408,#34635,.T.);
#55834=EDGE_CURVE('',#42410,#42409,#6379,.T.);
#55835=EDGE_CURVE('',#42381,#42410,#6380,.T.);
#55836=EDGE_CURVE('',#42411,#42412,#6381,.T.);
#55837=EDGE_CURVE('',#42382,#42411,#6382,.T.);
#55838=EDGE_CURVE('',#42413,#42383,#6383,.T.);
#55839=EDGE_CURVE('',#42414,#42413,#6384,.T.);
#55840=EDGE_CURVE('',#42412,#42414,#34636,.T.);
#55841=EDGE_CURVE('',#42415,#42416,#6385,.T.);
#55842=EDGE_CURVE('',#42384,#42415,#6386,.T.);
#55843=EDGE_CURVE('',#42417,#42385,#6387,.T.);
#55844=EDGE_CURVE('',#42418,#42417,#6388,.T.);
#55845=EDGE_CURVE('',#42416,#42418,#34637,.T.);
#55846=EDGE_CURVE('',#42419,#42420,#6389,.T.);
#55847=EDGE_CURVE('',#42386,#42419,#6390,.T.);
#55848=EDGE_CURVE('',#42421,#42387,#6391,.T.);
#55849=EDGE_CURVE('',#42422,#42421,#6392,.T.);
#55850=EDGE_CURVE('',#42420,#42422,#34638,.T.);
#55851=EDGE_CURVE('',#42423,#42258,#6393,.T.);
#55852=EDGE_CURVE('',#42424,#42423,#34639,.T.);
#55853=EDGE_CURVE('',#42425,#42424,#6394,.T.);
#55854=EDGE_CURVE('',#42388,#42425,#6395,.T.);
#55855=EDGE_CURVE('',#42426,#42427,#6396,.T.);
#55856=EDGE_CURVE('',#42389,#42426,#6397,.T.);
#55857=EDGE_CURVE('',#42428,#42390,#6398,.T.);
#55858=EDGE_CURVE('',#42429,#42428,#6399,.T.);
#55859=EDGE_CURVE('',#42427,#42429,#34640,.T.);
#55860=EDGE_CURVE('',#42430,#42391,#6400,.T.);
#55861=EDGE_CURVE('',#42431,#42430,#6401,.T.);
#55862=EDGE_CURVE('',#42432,#42431,#34641,.T.);
#55863=EDGE_CURVE('',#42433,#42432,#6402,.T.);
#55864=EDGE_CURVE('',#42392,#42433,#6403,.T.);
#55865=EDGE_CURVE('',#42265,#42393,#6404,.T.);
#55866=EDGE_CURVE('',#42272,#42264,#34642,.T.);
#55867=EDGE_CURVE('',#42394,#42271,#6405,.T.);
#55868=EDGE_CURVE('',#42395,#42262,#6406,.T.);
#55869=EDGE_CURVE('',#42434,#42396,#6407,.T.);
#55870=EDGE_CURVE('',#42435,#42434,#6408,.T.);
#55871=EDGE_CURVE('',#42263,#42435,#34643,.T.);
#55872=EDGE_CURVE('',#42274,#42397,#6409,.T.);
#55873=EDGE_CURVE('',#42304,#42273,#34644,.T.);
#55874=EDGE_CURVE('',#42398,#42303,#6410,.T.);
#55875=EDGE_CURVE('',#42282,#42399,#6411,.T.);
#55876=EDGE_CURVE('',#42289,#42281,#34645,.T.);
#55877=EDGE_CURVE('',#42400,#42288,#6412,.T.);
#55878=EDGE_CURVE('',#42401,#42279,#6413,.T.);
#55879=EDGE_CURVE('',#42298,#42402,#6414,.T.);
#55880=EDGE_CURVE('',#42280,#42297,#34646,.T.);
#55881=EDGE_CURVE('',#42291,#42403,#6415,.T.);
#55882=EDGE_CURVE('',#42436,#42290,#34647,.T.);
#55883=EDGE_CURVE('',#42437,#42436,#6416,.T.);
#55884=EDGE_CURVE('',#42404,#42437,#6417,.T.);
#55885=EDGE_CURVE('',#42405,#42295,#6418,.T.);
#55886=EDGE_CURVE('',#42306,#42406,#6419,.T.);
#55887=EDGE_CURVE('',#42296,#42305,#34648,.T.);
#55888=EDGE_CURVE('',#42328,#42308,#6420,.T.);
#55889=EDGE_CURVE('',#42438,#42327,#6421,.T.);
#55890=EDGE_CURVE('',#42439,#42438,#6422,.T.);
#55891=EDGE_CURVE('',#42309,#42439,#34649,.T.);
#55892=EDGE_CURVE('',#42440,#42439,#24256,.T.);
#55893=EDGE_CURVE('',#42310,#42440,#34650,.T.);
#55894=EDGE_CURVE('',#42311,#42441,#6423,.T.);
#55895=EDGE_CURVE('',#42442,#42440,#6424,.T.);
#55896=EDGE_CURVE('',#42443,#42442,#6425,.T.);
#55897=EDGE_CURVE('',#42441,#42443,#34651,.T.);
#55898=EDGE_CURVE('',#42412,#42408,#34652,.T.);
#55899=EDGE_CURVE('',#42416,#42414,#34653,.T.);
#55900=EDGE_CURVE('',#42420,#42418,#34654,.T.);
#55901=EDGE_CURVE('',#42441,#42422,#34655,.T.);
#55902=EDGE_CURVE('',#42436,#42443,#34656,.T.);
#55903=EDGE_CURVE('',#42432,#42435,#34657,.T.);
#55904=EDGE_CURVE('',#42424,#42431,#34658,.T.);
#55905=EDGE_CURVE('',#42427,#42423,#34659,.T.);
#55906=EDGE_CURVE('',#42409,#42429,#34660,.T.);
#55907=EDGE_CURVE('',#42438,#42442,#24257,.T.);
#55908=EDGE_CURVE('',#42377,#42437,#24258,.T.);
#55909=EDGE_CURVE('',#42351,#42421,#24259,.T.);
#55910=EDGE_CURVE('',#42366,#42434,#24260,.T.);
#55911=EDGE_CURVE('',#42363,#42433,#24261,.T.);
#55912=EDGE_CURVE('',#42357,#42428,#24262,.T.);
#55913=EDGE_CURVE('',#42341,#42410,#24263,.T.);
#55914=EDGE_CURVE('',#42361,#42430,#24264,.T.);
#55915=EDGE_CURVE('',#42355,#42425,#24265,.T.);
#55916=EDGE_CURVE('',#42356,#42426,#24266,.T.);
#55917=EDGE_CURVE('',#42347,#42417,#24267,.T.);
#55918=EDGE_CURVE('',#42350,#42419,#24268,.T.);
#55919=EDGE_CURVE('',#42343,#42413,#24269,.T.);
#55920=EDGE_CURVE('',#42346,#42415,#24270,.T.);
#55921=EDGE_CURVE('',#42339,#42407,#24271,.T.);
#55922=EDGE_CURVE('',#42342,#42411,#24272,.T.);
#55923=EDGE_CURVE('',#42335,#42337,#24273,.T.);
#55924=EDGE_CURVE('',#42334,#42336,#24274,.T.);
#55925=EDGE_CURVE('',#42444,#42444,#34661,.T.);
#55926=EDGE_CURVE('',#42444,#42445,#24275,.T.);
#55927=EDGE_CURVE('',#42445,#42445,#34662,.T.);
#55928=EDGE_CURVE('',#42446,#42447,#34663,.T.);
#55929=EDGE_CURVE('',#42446,#42448,#24276,.T.);
#55930=EDGE_CURVE('',#42449,#42448,#34664,.T.);
#55931=EDGE_CURVE('',#42447,#42449,#24277,.T.);
#55932=EDGE_CURVE('',#42450,#42446,#24278,.T.);
#55933=EDGE_CURVE('',#42450,#42451,#24279,.T.);
#55934=EDGE_CURVE('',#42448,#42451,#24280,.T.);
#55935=EDGE_CURVE('',#42452,#42450,#24281,.T.);
#55936=EDGE_CURVE('',#42452,#42453,#24282,.T.);
#55937=EDGE_CURVE('',#42451,#42453,#24283,.T.);
#55938=EDGE_CURVE('',#42447,#42452,#24284,.T.);
#55939=EDGE_CURVE('',#42453,#42449,#24285,.T.);
#81717=ORIENTED_EDGE('',*,*,#55638,.F.);
#81718=ORIENTED_EDGE('',*,*,#55639,.T.);
#81719=ORIENTED_EDGE('',*,*,#55640,.F.);
#81720=ORIENTED_EDGE('',*,*,#55639,.F.);
#81721=ORIENTED_EDGE('',*,*,#55640,.T.);
#81722=ORIENTED_EDGE('',*,*,#55641,.T.);
#81723=ORIENTED_EDGE('',*,*,#55642,.F.);
#81724=ORIENTED_EDGE('',*,*,#55641,.F.);
#81725=ORIENTED_EDGE('',*,*,#55643,.T.);
#81726=ORIENTED_EDGE('',*,*,#55644,.T.);
#81727=ORIENTED_EDGE('',*,*,#55645,.T.);
#81728=ORIENTED_EDGE('',*,*,#55646,.T.);
#81729=ORIENTED_EDGE('',*,*,#55647,.T.);
#81730=ORIENTED_EDGE('',*,*,#55648,.T.);
#81731=ORIENTED_EDGE('',*,*,#55649,.T.);
#81732=ORIENTED_EDGE('',*,*,#55650,.T.);
#81733=ORIENTED_EDGE('',*,*,#55651,.T.);
#81734=ORIENTED_EDGE('',*,*,#55652,.F.);
#81735=ORIENTED_EDGE('',*,*,#55653,.T.);
#81736=ORIENTED_EDGE('',*,*,#55654,.T.);
#81737=ORIENTED_EDGE('',*,*,#55655,.T.);
#81738=ORIENTED_EDGE('',*,*,#55656,.T.);
#81739=ORIENTED_EDGE('',*,*,#55657,.T.);
#81740=ORIENTED_EDGE('',*,*,#55658,.T.);
#81741=ORIENTED_EDGE('',*,*,#55659,.T.);
#81742=ORIENTED_EDGE('',*,*,#55660,.T.);
#81743=ORIENTED_EDGE('',*,*,#55661,.F.);
#81744=ORIENTED_EDGE('',*,*,#55662,.T.);
#81745=ORIENTED_EDGE('',*,*,#55663,.T.);
#81746=ORIENTED_EDGE('',*,*,#55664,.T.);
#81747=ORIENTED_EDGE('',*,*,#55665,.T.);
#81748=ORIENTED_EDGE('',*,*,#55666,.T.);
#81749=ORIENTED_EDGE('',*,*,#55667,.T.);
#81750=ORIENTED_EDGE('',*,*,#55668,.T.);
#81751=ORIENTED_EDGE('',*,*,#55669,.F.);
#81752=ORIENTED_EDGE('',*,*,#55670,.T.);
#81753=ORIENTED_EDGE('',*,*,#55671,.T.);
#81754=ORIENTED_EDGE('',*,*,#55672,.T.);
#81755=ORIENTED_EDGE('',*,*,#55673,.T.);
#81756=ORIENTED_EDGE('',*,*,#55674,.T.);
#81757=ORIENTED_EDGE('',*,*,#55675,.T.);
#81758=ORIENTED_EDGE('',*,*,#55676,.T.);
#81759=ORIENTED_EDGE('',*,*,#55677,.T.);
#81760=ORIENTED_EDGE('',*,*,#55678,.F.);
#81761=ORIENTED_EDGE('',*,*,#55679,.T.);
#81762=ORIENTED_EDGE('',*,*,#55680,.T.);
#81763=ORIENTED_EDGE('',*,*,#55681,.T.);
#81764=ORIENTED_EDGE('',*,*,#55682,.T.);
#81765=ORIENTED_EDGE('',*,*,#55683,.T.);
#81766=ORIENTED_EDGE('',*,*,#55684,.T.);
#81767=ORIENTED_EDGE('',*,*,#55685,.F.);
#81768=ORIENTED_EDGE('',*,*,#55686,.T.);
#81769=ORIENTED_EDGE('',*,*,#55687,.T.);
#81770=ORIENTED_EDGE('',*,*,#55688,.T.);
#81771=ORIENTED_EDGE('',*,*,#55689,.T.);
#81772=ORIENTED_EDGE('',*,*,#55690,.T.);
#81773=ORIENTED_EDGE('',*,*,#55691,.T.);
#81774=ORIENTED_EDGE('',*,*,#55692,.T.);
#81775=ORIENTED_EDGE('',*,*,#55693,.F.);
#81776=ORIENTED_EDGE('',*,*,#55694,.T.);
#81777=ORIENTED_EDGE('',*,*,#55695,.T.);
#81778=ORIENTED_EDGE('',*,*,#55696,.T.);
#81779=ORIENTED_EDGE('',*,*,#55697,.T.);
#81780=ORIENTED_EDGE('',*,*,#55698,.F.);
#81781=ORIENTED_EDGE('',*,*,#55699,.T.);
#81782=ORIENTED_EDGE('',*,*,#55700,.T.);
#81783=ORIENTED_EDGE('',*,*,#55701,.F.);
#81784=ORIENTED_EDGE('',*,*,#55702,.T.);
#81785=ORIENTED_EDGE('',*,*,#55703,.F.);
#81786=ORIENTED_EDGE('',*,*,#55704,.F.);
#81787=ORIENTED_EDGE('',*,*,#55705,.F.);
#81788=ORIENTED_EDGE('',*,*,#55706,.F.);
#81789=ORIENTED_EDGE('',*,*,#55707,.F.);
#81790=ORIENTED_EDGE('',*,*,#55708,.F.);
#81791=ORIENTED_EDGE('',*,*,#55709,.F.);
#81792=ORIENTED_EDGE('',*,*,#55710,.F.);
#81793=ORIENTED_EDGE('',*,*,#55711,.F.);
#81794=ORIENTED_EDGE('',*,*,#55712,.F.);
#81795=ORIENTED_EDGE('',*,*,#55654,.F.);
#81796=ORIENTED_EDGE('',*,*,#55713,.F.);
#81797=ORIENTED_EDGE('',*,*,#55655,.F.);
#81798=ORIENTED_EDGE('',*,*,#55714,.F.);
#81799=ORIENTED_EDGE('',*,*,#55687,.F.);
#81800=ORIENTED_EDGE('',*,*,#55715,.F.);
#81801=ORIENTED_EDGE('',*,*,#55679,.F.);
#81802=ORIENTED_EDGE('',*,*,#55716,.F.);
#81803=ORIENTED_EDGE('',*,*,#55663,.F.);
#81804=ORIENTED_EDGE('',*,*,#55717,.F.);
#81805=ORIENTED_EDGE('',*,*,#55672,.F.);
#81806=ORIENTED_EDGE('',*,*,#55718,.F.);
#81807=ORIENTED_EDGE('',*,*,#55719,.F.);
#81808=ORIENTED_EDGE('',*,*,#55720,.F.);
#81809=ORIENTED_EDGE('',*,*,#55721,.F.);
#81810=ORIENTED_EDGE('',*,*,#55722,.F.);
#81811=ORIENTED_EDGE('',*,*,#55723,.F.);
#81812=ORIENTED_EDGE('',*,*,#55724,.F.);
#81813=ORIENTED_EDGE('',*,*,#55725,.F.);
#81814=ORIENTED_EDGE('',*,*,#55726,.F.);
#81815=ORIENTED_EDGE('',*,*,#55727,.F.);
#81816=ORIENTED_EDGE('',*,*,#55699,.F.);
#81817=ORIENTED_EDGE('',*,*,#55728,.F.);
#81818=ORIENTED_EDGE('',*,*,#55729,.F.);
#81819=ORIENTED_EDGE('',*,*,#55642,.T.);
#81820=ORIENTED_EDGE('',*,*,#55701,.T.);
#81821=ORIENTED_EDGE('',*,*,#55730,.T.);
#81822=ORIENTED_EDGE('',*,*,#55731,.T.);
#81823=ORIENTED_EDGE('',*,*,#55732,.T.);
#81824=ORIENTED_EDGE('',*,*,#55733,.F.);
#81825=ORIENTED_EDGE('',*,*,#55734,.F.);
#81826=ORIENTED_EDGE('',*,*,#55735,.F.);
#81827=ORIENTED_EDGE('',*,*,#55736,.F.);
#81828=ORIENTED_EDGE('',*,*,#55704,.T.);
#81829=ORIENTED_EDGE('',*,*,#55737,.F.);
#81830=ORIENTED_EDGE('',*,*,#55738,.F.);
#81831=ORIENTED_EDGE('',*,*,#55726,.T.);
#81832=ORIENTED_EDGE('',*,*,#55739,.F.);
#81833=ORIENTED_EDGE('',*,*,#55740,.F.);
#81834=ORIENTED_EDGE('',*,*,#55741,.F.);
#81835=ORIENTED_EDGE('',*,*,#55742,.F.);
#81836=ORIENTED_EDGE('',*,*,#55743,.F.);
#81837=ORIENTED_EDGE('',*,*,#55724,.T.);
#81838=ORIENTED_EDGE('',*,*,#55744,.F.);
#81839=ORIENTED_EDGE('',*,*,#55745,.F.);
#81840=ORIENTED_EDGE('',*,*,#55746,.F.);
#81841=ORIENTED_EDGE('',*,*,#55747,.F.);
#81842=ORIENTED_EDGE('',*,*,#55748,.F.);
#81843=ORIENTED_EDGE('',*,*,#55722,.T.);
#81844=ORIENTED_EDGE('',*,*,#55749,.F.);
#81845=ORIENTED_EDGE('',*,*,#55750,.F.);
#81846=ORIENTED_EDGE('',*,*,#55751,.F.);
#81847=ORIENTED_EDGE('',*,*,#55752,.F.);
#81848=ORIENTED_EDGE('',*,*,#55643,.F.);
#81849=ORIENTED_EDGE('',*,*,#55753,.F.);
#81850=ORIENTED_EDGE('',*,*,#55754,.F.);
#81851=ORIENTED_EDGE('',*,*,#55755,.F.);
#81852=ORIENTED_EDGE('',*,*,#55708,.T.);
#81853=ORIENTED_EDGE('',*,*,#55756,.F.);
#81854=ORIENTED_EDGE('',*,*,#55757,.F.);
#81855=ORIENTED_EDGE('',*,*,#55706,.T.);
#81856=ORIENTED_EDGE('',*,*,#55758,.F.);
#81857=ORIENTED_EDGE('',*,*,#55759,.F.);
#81858=ORIENTED_EDGE('',*,*,#55760,.F.);
#81859=ORIENTED_EDGE('',*,*,#55761,.F.);
#81860=ORIENTED_EDGE('',*,*,#55762,.F.);
#81861=ORIENTED_EDGE('',*,*,#55763,.F.);
#81862=ORIENTED_EDGE('',*,*,#55764,.F.);
#81863=ORIENTED_EDGE('',*,*,#55765,.F.);
#81864=ORIENTED_EDGE('',*,*,#55710,.T.);
#81865=ORIENTED_EDGE('',*,*,#55766,.F.);
#81866=ORIENTED_EDGE('',*,*,#55767,.F.);
#81867=ORIENTED_EDGE('',*,*,#55768,.F.);
#81868=ORIENTED_EDGE('',*,*,#55769,.F.);
#81869=ORIENTED_EDGE('',*,*,#55656,.F.);
#81870=ORIENTED_EDGE('',*,*,#55713,.T.);
#81871=ORIENTED_EDGE('',*,*,#55653,.F.);
#81872=ORIENTED_EDGE('',*,*,#55647,.F.);
#81873=ORIENTED_EDGE('',*,*,#55712,.T.);
#81874=ORIENTED_EDGE('',*,*,#55770,.F.);
#81875=ORIENTED_EDGE('',*,*,#55771,.F.);
#81876=ORIENTED_EDGE('',*,*,#55772,.F.);
#81877=ORIENTED_EDGE('',*,*,#55773,.F.);
#81878=ORIENTED_EDGE('',*,*,#55774,.F.);
#81879=ORIENTED_EDGE('',*,*,#55775,.F.);
#81880=ORIENTED_EDGE('',*,*,#55776,.F.);
#81881=ORIENTED_EDGE('',*,*,#55688,.F.);
#81882=ORIENTED_EDGE('',*,*,#55714,.T.);
#81883=ORIENTED_EDGE('',*,*,#55662,.F.);
#81884=ORIENTED_EDGE('',*,*,#55777,.F.);
#81885=ORIENTED_EDGE('',*,*,#55778,.F.);
#81886=ORIENTED_EDGE('',*,*,#55779,.F.);
#81887=ORIENTED_EDGE('',*,*,#55673,.F.);
#81888=ORIENTED_EDGE('',*,*,#55717,.T.);
#81889=ORIENTED_EDGE('',*,*,#55670,.F.);
#81890=ORIENTED_EDGE('',*,*,#55664,.F.);
#81891=ORIENTED_EDGE('',*,*,#55716,.T.);
#81892=ORIENTED_EDGE('',*,*,#55686,.F.);
#81893=ORIENTED_EDGE('',*,*,#55780,.F.);
#81894=ORIENTED_EDGE('',*,*,#55781,.F.);
#81895=ORIENTED_EDGE('',*,*,#55782,.F.);
#81896=ORIENTED_EDGE('',*,*,#55783,.F.);
#81897=ORIENTED_EDGE('',*,*,#55784,.F.);
#81898=ORIENTED_EDGE('',*,*,#55785,.F.);
#81899=ORIENTED_EDGE('',*,*,#55786,.F.);
#81900=ORIENTED_EDGE('',*,*,#55718,.T.);
#81901=ORIENTED_EDGE('',*,*,#55671,.F.);
#81902=ORIENTED_EDGE('',*,*,#55680,.F.);
#81903=ORIENTED_EDGE('',*,*,#55715,.T.);
#81904=ORIENTED_EDGE('',*,*,#55694,.F.);
#81905=ORIENTED_EDGE('',*,*,#55787,.F.);
#81906=ORIENTED_EDGE('',*,*,#55788,.F.);
#81907=ORIENTED_EDGE('',*,*,#55789,.F.);
#81908=ORIENTED_EDGE('',*,*,#55790,.F.);
#81909=ORIENTED_EDGE('',*,*,#55791,.F.);
#81910=ORIENTED_EDGE('',*,*,#55792,.F.);
#81911=ORIENTED_EDGE('',*,*,#55734,.T.);
#81912=ORIENTED_EDGE('',*,*,#55793,.F.);
#81913=ORIENTED_EDGE('',*,*,#55741,.T.);
#81914=ORIENTED_EDGE('',*,*,#55794,.F.);
#81915=ORIENTED_EDGE('',*,*,#55795,.F.);
#81916=ORIENTED_EDGE('',*,*,#55796,.F.);
#81917=ORIENTED_EDGE('',*,*,#55746,.T.);
#81918=ORIENTED_EDGE('',*,*,#55797,.F.);
#81919=ORIENTED_EDGE('',*,*,#55798,.F.);
#81920=ORIENTED_EDGE('',*,*,#55799,.F.);
#81921=ORIENTED_EDGE('',*,*,#55751,.T.);
#81922=ORIENTED_EDGE('',*,*,#55800,.F.);
#81923=ORIENTED_EDGE('',*,*,#55801,.F.);
#81924=ORIENTED_EDGE('',*,*,#55646,.F.);
#81925=ORIENTED_EDGE('',*,*,#55802,.F.);
#81926=ORIENTED_EDGE('',*,*,#55803,.F.);
#81927=ORIENTED_EDGE('',*,*,#55753,.T.);
#81928=ORIENTED_EDGE('',*,*,#55804,.F.);
#81929=ORIENTED_EDGE('',*,*,#55760,.T.);
#81930=ORIENTED_EDGE('',*,*,#55805,.F.);
#81931=ORIENTED_EDGE('',*,*,#55806,.F.);
#81932=ORIENTED_EDGE('',*,*,#55807,.F.);
#81933=ORIENTED_EDGE('',*,*,#55808,.F.);
#81934=ORIENTED_EDGE('',*,*,#55809,.F.);
#81935=ORIENTED_EDGE('',*,*,#55763,.T.);
#81936=ORIENTED_EDGE('',*,*,#55810,.F.);
#81937=ORIENTED_EDGE('',*,*,#55811,.F.);
#81938=ORIENTED_EDGE('',*,*,#55812,.F.);
#81939=ORIENTED_EDGE('',*,*,#55768,.T.);
#81940=ORIENTED_EDGE('',*,*,#55813,.F.);
#81941=ORIENTED_EDGE('',*,*,#55772,.T.);
#81942=ORIENTED_EDGE('',*,*,#55814,.F.);
#81943=ORIENTED_EDGE('',*,*,#55815,.F.);
#81944=ORIENTED_EDGE('',*,*,#55816,.F.);
#81945=ORIENTED_EDGE('',*,*,#55817,.F.);
#81946=ORIENTED_EDGE('',*,*,#55818,.F.);
#81947=ORIENTED_EDGE('',*,*,#55775,.T.);
#81948=ORIENTED_EDGE('',*,*,#55819,.F.);
#81949=ORIENTED_EDGE('',*,*,#55820,.F.);
#81950=ORIENTED_EDGE('',*,*,#55821,.F.);
#81951=ORIENTED_EDGE('',*,*,#55778,.T.);
#81952=ORIENTED_EDGE('',*,*,#55822,.F.);
#81953=ORIENTED_EDGE('',*,*,#55781,.T.);
#81954=ORIENTED_EDGE('',*,*,#55823,.F.);
#81955=ORIENTED_EDGE('',*,*,#55824,.F.);
#81956=ORIENTED_EDGE('',*,*,#55825,.F.);
#81957=ORIENTED_EDGE('',*,*,#55826,.F.);
#81958=ORIENTED_EDGE('',*,*,#55827,.F.);
#81959=ORIENTED_EDGE('',*,*,#55784,.T.);
#81960=ORIENTED_EDGE('',*,*,#55828,.F.);
#81961=ORIENTED_EDGE('',*,*,#55788,.T.);
#81962=ORIENTED_EDGE('',*,*,#55829,.F.);
#81963=ORIENTED_EDGE('',*,*,#55830,.F.);
#81964=ORIENTED_EDGE('',*,*,#55831,.F.);
#81965=ORIENTED_EDGE('',*,*,#55832,.F.);
#81966=ORIENTED_EDGE('',*,*,#55833,.F.);
#81967=ORIENTED_EDGE('',*,*,#55834,.F.);
#81968=ORIENTED_EDGE('',*,*,#55835,.F.);
#81969=ORIENTED_EDGE('',*,*,#55791,.T.);
#81970=ORIENTED_EDGE('',*,*,#55836,.F.);
#81971=ORIENTED_EDGE('',*,*,#55837,.F.);
#81972=ORIENTED_EDGE('',*,*,#55795,.T.);
#81973=ORIENTED_EDGE('',*,*,#55838,.F.);
#81974=ORIENTED_EDGE('',*,*,#55839,.F.);
#81975=ORIENTED_EDGE('',*,*,#55840,.F.);
#81976=ORIENTED_EDGE('',*,*,#55841,.F.);
#81977=ORIENTED_EDGE('',*,*,#55842,.F.);
#81978=ORIENTED_EDGE('',*,*,#55798,.T.);
#81979=ORIENTED_EDGE('',*,*,#55843,.F.);
#81980=ORIENTED_EDGE('',*,*,#55844,.F.);
#81981=ORIENTED_EDGE('',*,*,#55845,.F.);
#81982=ORIENTED_EDGE('',*,*,#55846,.F.);
#81983=ORIENTED_EDGE('',*,*,#55847,.F.);
#81984=ORIENTED_EDGE('',*,*,#55801,.T.);
#81985=ORIENTED_EDGE('',*,*,#55848,.F.);
#81986=ORIENTED_EDGE('',*,*,#55849,.F.);
#81987=ORIENTED_EDGE('',*,*,#55850,.F.);
#81988=ORIENTED_EDGE('',*,*,#55645,.F.);
#81989=ORIENTED_EDGE('',*,*,#55851,.F.);
#81990=ORIENTED_EDGE('',*,*,#55852,.F.);
#81991=ORIENTED_EDGE('',*,*,#55853,.F.);
#81992=ORIENTED_EDGE('',*,*,#55854,.F.);
#81993=ORIENTED_EDGE('',*,*,#55802,.T.);
#81994=ORIENTED_EDGE('',*,*,#55855,.F.);
#81995=ORIENTED_EDGE('',*,*,#55856,.F.);
#81996=ORIENTED_EDGE('',*,*,#55806,.T.);
#81997=ORIENTED_EDGE('',*,*,#55857,.F.);
#81998=ORIENTED_EDGE('',*,*,#55858,.F.);
#81999=ORIENTED_EDGE('',*,*,#55859,.F.);
#82000=ORIENTED_EDGE('',*,*,#55860,.F.);
#82001=ORIENTED_EDGE('',*,*,#55861,.F.);
#82002=ORIENTED_EDGE('',*,*,#55862,.F.);
#82003=ORIENTED_EDGE('',*,*,#55863,.F.);
#82004=ORIENTED_EDGE('',*,*,#55864,.F.);
#82005=ORIENTED_EDGE('',*,*,#55808,.T.);
#82006=ORIENTED_EDGE('',*,*,#55865,.F.);
#82007=ORIENTED_EDGE('',*,*,#55651,.F.);
#82008=ORIENTED_EDGE('',*,*,#55866,.F.);
#82009=ORIENTED_EDGE('',*,*,#55658,.F.);
#82010=ORIENTED_EDGE('',*,*,#55867,.F.);
#82011=ORIENTED_EDGE('',*,*,#55811,.T.);
#82012=ORIENTED_EDGE('',*,*,#55649,.F.);
#82013=ORIENTED_EDGE('',*,*,#55868,.F.);
#82014=ORIENTED_EDGE('',*,*,#55815,.T.);
#82015=ORIENTED_EDGE('',*,*,#55869,.F.);
#82016=ORIENTED_EDGE('',*,*,#55870,.F.);
#82017=ORIENTED_EDGE('',*,*,#55871,.F.);
#82018=ORIENTED_EDGE('',*,*,#55872,.F.);
#82019=ORIENTED_EDGE('',*,*,#55660,.F.);
#82020=ORIENTED_EDGE('',*,*,#55873,.F.);
#82021=ORIENTED_EDGE('',*,*,#55690,.F.);
#82022=ORIENTED_EDGE('',*,*,#55874,.F.);
#82023=ORIENTED_EDGE('',*,*,#55817,.T.);
#82024=ORIENTED_EDGE('',*,*,#55875,.F.);
#82025=ORIENTED_EDGE('',*,*,#55668,.F.);
#82026=ORIENTED_EDGE('',*,*,#55876,.F.);
#82027=ORIENTED_EDGE('',*,*,#55675,.F.);
#82028=ORIENTED_EDGE('',*,*,#55877,.F.);
#82029=ORIENTED_EDGE('',*,*,#55820,.T.);
#82030=ORIENTED_EDGE('',*,*,#55666,.F.);
#82031=ORIENTED_EDGE('',*,*,#55878,.F.);
#82032=ORIENTED_EDGE('',*,*,#55824,.T.);
#82033=ORIENTED_EDGE('',*,*,#55879,.F.);
#82034=ORIENTED_EDGE('',*,*,#55684,.F.);
#82035=ORIENTED_EDGE('',*,*,#55880,.F.);
#82036=ORIENTED_EDGE('',*,*,#55881,.F.);
#82037=ORIENTED_EDGE('',*,*,#55677,.F.);
#82038=ORIENTED_EDGE('',*,*,#55882,.F.);
#82039=ORIENTED_EDGE('',*,*,#55883,.F.);
#82040=ORIENTED_EDGE('',*,*,#55884,.F.);
#82041=ORIENTED_EDGE('',*,*,#55826,.T.);
#82042=ORIENTED_EDGE('',*,*,#55682,.F.);
#82043=ORIENTED_EDGE('',*,*,#55885,.F.);
#82044=ORIENTED_EDGE('',*,*,#55830,.T.);
#82045=ORIENTED_EDGE('',*,*,#55886,.F.);
#82046=ORIENTED_EDGE('',*,*,#55692,.F.);
#82047=ORIENTED_EDGE('',*,*,#55887,.F.);
#82048=ORIENTED_EDGE('',*,*,#55888,.F.);
#82049=ORIENTED_EDGE('',*,*,#55720,.T.);
#82050=ORIENTED_EDGE('',*,*,#55889,.F.);
#82051=ORIENTED_EDGE('',*,*,#55890,.F.);
#82052=ORIENTED_EDGE('',*,*,#55891,.F.);
#82053=ORIENTED_EDGE('',*,*,#55695,.F.);
#82054=ORIENTED_EDGE('',*,*,#55696,.F.);
#82055=ORIENTED_EDGE('',*,*,#55891,.T.);
#82056=ORIENTED_EDGE('',*,*,#55892,.F.);
#82057=ORIENTED_EDGE('',*,*,#55893,.F.);
#82058=ORIENTED_EDGE('',*,*,#55894,.F.);
#82059=ORIENTED_EDGE('',*,*,#55697,.F.);
#82060=ORIENTED_EDGE('',*,*,#55893,.T.);
#82061=ORIENTED_EDGE('',*,*,#55895,.F.);
#82062=ORIENTED_EDGE('',*,*,#55896,.F.);
#82063=ORIENTED_EDGE('',*,*,#55897,.F.);
#82064=ORIENTED_EDGE('',*,*,#55898,.F.);
#82065=ORIENTED_EDGE('',*,*,#55840,.T.);
#82066=ORIENTED_EDGE('',*,*,#55899,.F.);
#82067=ORIENTED_EDGE('',*,*,#55845,.T.);
#82068=ORIENTED_EDGE('',*,*,#55900,.F.);
#82069=ORIENTED_EDGE('',*,*,#55850,.T.);
#82070=ORIENTED_EDGE('',*,*,#55901,.F.);
#82071=ORIENTED_EDGE('',*,*,#55897,.T.);
#82072=ORIENTED_EDGE('',*,*,#55902,.F.);
#82073=ORIENTED_EDGE('',*,*,#55882,.T.);
#82074=ORIENTED_EDGE('',*,*,#55676,.F.);
#82075=ORIENTED_EDGE('',*,*,#55876,.T.);
#82076=ORIENTED_EDGE('',*,*,#55667,.F.);
#82077=ORIENTED_EDGE('',*,*,#55880,.T.);
#82078=ORIENTED_EDGE('',*,*,#55683,.F.);
#82079=ORIENTED_EDGE('',*,*,#55887,.T.);
#82080=ORIENTED_EDGE('',*,*,#55691,.F.);
#82081=ORIENTED_EDGE('',*,*,#55873,.T.);
#82082=ORIENTED_EDGE('',*,*,#55659,.F.);
#82083=ORIENTED_EDGE('',*,*,#55866,.T.);
#82084=ORIENTED_EDGE('',*,*,#55650,.F.);
#82085=ORIENTED_EDGE('',*,*,#55871,.T.);
#82086=ORIENTED_EDGE('',*,*,#55903,.F.);
#82087=ORIENTED_EDGE('',*,*,#55862,.T.);
#82088=ORIENTED_EDGE('',*,*,#55904,.F.);
#82089=ORIENTED_EDGE('',*,*,#55852,.T.);
#82090=ORIENTED_EDGE('',*,*,#55905,.F.);
#82091=ORIENTED_EDGE('',*,*,#55859,.T.);
#82092=ORIENTED_EDGE('',*,*,#55906,.F.);
#82093=ORIENTED_EDGE('',*,*,#55833,.T.);
#82094=ORIENTED_EDGE('',*,*,#55638,.T.);
#82095=ORIENTED_EDGE('',*,*,#55890,.T.);
#82096=ORIENTED_EDGE('',*,*,#55907,.T.);
#82097=ORIENTED_EDGE('',*,*,#55895,.T.);
#82098=ORIENTED_EDGE('',*,*,#55892,.T.);
#82099=ORIENTED_EDGE('',*,*,#55785,.T.);
#82100=ORIENTED_EDGE('',*,*,#55827,.T.);
#82101=ORIENTED_EDGE('',*,*,#55884,.T.);
#82102=ORIENTED_EDGE('',*,*,#55908,.F.);
#82103=ORIENTED_EDGE('',*,*,#55889,.T.);
#82104=ORIENTED_EDGE('',*,*,#55719,.T.);
#82105=ORIENTED_EDGE('',*,*,#55786,.T.);
#82106=ORIENTED_EDGE('',*,*,#55908,.T.);
#82107=ORIENTED_EDGE('',*,*,#55883,.T.);
#82108=ORIENTED_EDGE('',*,*,#55902,.T.);
#82109=ORIENTED_EDGE('',*,*,#55896,.T.);
#82110=ORIENTED_EDGE('',*,*,#55907,.F.);
#82111=ORIENTED_EDGE('',*,*,#55750,.T.);
#82112=ORIENTED_EDGE('',*,*,#55909,.T.);
#82113=ORIENTED_EDGE('',*,*,#55848,.T.);
#82114=ORIENTED_EDGE('',*,*,#55800,.T.);
#82115=ORIENTED_EDGE('',*,*,#55749,.T.);
#82116=ORIENTED_EDGE('',*,*,#55721,.T.);
#82117=ORIENTED_EDGE('',*,*,#55888,.T.);
#82118=ORIENTED_EDGE('',*,*,#55698,.T.);
#82119=ORIENTED_EDGE('',*,*,#55894,.T.);
#82120=ORIENTED_EDGE('',*,*,#55901,.T.);
#82121=ORIENTED_EDGE('',*,*,#55849,.T.);
#82122=ORIENTED_EDGE('',*,*,#55909,.F.);
#82123=ORIENTED_EDGE('',*,*,#55787,.T.);
#82124=ORIENTED_EDGE('',*,*,#55693,.T.);
#82125=ORIENTED_EDGE('',*,*,#55886,.T.);
#82126=ORIENTED_EDGE('',*,*,#55829,.T.);
#82127=ORIENTED_EDGE('',*,*,#55776,.T.);
#82128=ORIENTED_EDGE('',*,*,#55818,.T.);
#82129=ORIENTED_EDGE('',*,*,#55874,.T.);
#82130=ORIENTED_EDGE('',*,*,#55689,.F.);
#82131=ORIENTED_EDGE('',*,*,#55780,.T.);
#82132=ORIENTED_EDGE('',*,*,#55685,.T.);
#82133=ORIENTED_EDGE('',*,*,#55879,.T.);
#82134=ORIENTED_EDGE('',*,*,#55823,.T.);
#82135=ORIENTED_EDGE('',*,*,#55789,.T.);
#82136=ORIENTED_EDGE('',*,*,#55828,.T.);
#82137=ORIENTED_EDGE('',*,*,#55885,.T.);
#82138=ORIENTED_EDGE('',*,*,#55681,.F.);
#82139=ORIENTED_EDGE('',*,*,#55783,.T.);
#82140=ORIENTED_EDGE('',*,*,#55678,.T.);
#82141=ORIENTED_EDGE('',*,*,#55881,.T.);
#82142=ORIENTED_EDGE('',*,*,#55825,.T.);
#82143=ORIENTED_EDGE('',*,*,#55779,.T.);
#82144=ORIENTED_EDGE('',*,*,#55821,.T.);
#82145=ORIENTED_EDGE('',*,*,#55877,.T.);
#82146=ORIENTED_EDGE('',*,*,#55674,.F.);
#82147=ORIENTED_EDGE('',*,*,#55777,.T.);
#82148=ORIENTED_EDGE('',*,*,#55669,.T.);
#82149=ORIENTED_EDGE('',*,*,#55875,.T.);
#82150=ORIENTED_EDGE('',*,*,#55819,.T.);
#82151=ORIENTED_EDGE('',*,*,#55782,.T.);
#82152=ORIENTED_EDGE('',*,*,#55822,.T.);
#82153=ORIENTED_EDGE('',*,*,#55878,.T.);
#82154=ORIENTED_EDGE('',*,*,#55665,.F.);
#82155=ORIENTED_EDGE('',*,*,#55771,.T.);
#82156=ORIENTED_EDGE('',*,*,#55910,.T.);
#82157=ORIENTED_EDGE('',*,*,#55869,.T.);
#82158=ORIENTED_EDGE('',*,*,#55814,.T.);
#82159=ORIENTED_EDGE('',*,*,#55764,.T.);
#82160=ORIENTED_EDGE('',*,*,#55809,.T.);
#82161=ORIENTED_EDGE('',*,*,#55864,.T.);
#82162=ORIENTED_EDGE('',*,*,#55911,.F.);
#82163=ORIENTED_EDGE('',*,*,#55770,.T.);
#82164=ORIENTED_EDGE('',*,*,#55711,.T.);
#82165=ORIENTED_EDGE('',*,*,#55765,.T.);
#82166=ORIENTED_EDGE('',*,*,#55911,.T.);
#82167=ORIENTED_EDGE('',*,*,#55863,.T.);
#82168=ORIENTED_EDGE('',*,*,#55903,.T.);
#82169=ORIENTED_EDGE('',*,*,#55870,.T.);
#82170=ORIENTED_EDGE('',*,*,#55910,.F.);
#82171=ORIENTED_EDGE('',*,*,#55774,.T.);
#82172=ORIENTED_EDGE('',*,*,#55661,.T.);
#82173=ORIENTED_EDGE('',*,*,#55872,.T.);
#82174=ORIENTED_EDGE('',*,*,#55816,.T.);
#82175=ORIENTED_EDGE('',*,*,#55769,.T.);
#82176=ORIENTED_EDGE('',*,*,#55812,.T.);
#82177=ORIENTED_EDGE('',*,*,#55867,.T.);
#82178=ORIENTED_EDGE('',*,*,#55657,.F.);
#82179=ORIENTED_EDGE('',*,*,#55767,.T.);
#82180=ORIENTED_EDGE('',*,*,#55652,.T.);
#82181=ORIENTED_EDGE('',*,*,#55865,.T.);
#82182=ORIENTED_EDGE('',*,*,#55810,.T.);
#82183=ORIENTED_EDGE('',*,*,#55773,.T.);
#82184=ORIENTED_EDGE('',*,*,#55813,.T.);
#82185=ORIENTED_EDGE('',*,*,#55868,.T.);
#82186=ORIENTED_EDGE('',*,*,#55648,.F.);
#82187=ORIENTED_EDGE('',*,*,#55759,.T.);
#82188=ORIENTED_EDGE('',*,*,#55912,.T.);
#82189=ORIENTED_EDGE('',*,*,#55857,.T.);
#82190=ORIENTED_EDGE('',*,*,#55805,.T.);
#82191=ORIENTED_EDGE('',*,*,#55735,.T.);
#82192=ORIENTED_EDGE('',*,*,#55792,.T.);
#82193=ORIENTED_EDGE('',*,*,#55835,.T.);
#82194=ORIENTED_EDGE('',*,*,#55913,.F.);
#82195=ORIENTED_EDGE('',*,*,#55758,.T.);
#82196=ORIENTED_EDGE('',*,*,#55705,.T.);
#82197=ORIENTED_EDGE('',*,*,#55736,.T.);
#82198=ORIENTED_EDGE('',*,*,#55913,.T.);
#82199=ORIENTED_EDGE('',*,*,#55834,.T.);
#82200=ORIENTED_EDGE('',*,*,#55906,.T.);
#82201=ORIENTED_EDGE('',*,*,#55858,.T.);
#82202=ORIENTED_EDGE('',*,*,#55912,.F.);
#82203=ORIENTED_EDGE('',*,*,#55762,.T.);
#82204=ORIENTED_EDGE('',*,*,#55914,.T.);
#82205=ORIENTED_EDGE('',*,*,#55860,.T.);
#82206=ORIENTED_EDGE('',*,*,#55807,.T.);
#82207=ORIENTED_EDGE('',*,*,#55754,.T.);
#82208=ORIENTED_EDGE('',*,*,#55803,.T.);
#82209=ORIENTED_EDGE('',*,*,#55854,.T.);
#82210=ORIENTED_EDGE('',*,*,#55915,.F.);
#82211=ORIENTED_EDGE('',*,*,#55766,.T.);
#82212=ORIENTED_EDGE('',*,*,#55709,.T.);
#82213=ORIENTED_EDGE('',*,*,#55755,.T.);
#82214=ORIENTED_EDGE('',*,*,#55915,.T.);
#82215=ORIENTED_EDGE('',*,*,#55853,.T.);
#82216=ORIENTED_EDGE('',*,*,#55904,.T.);
#82217=ORIENTED_EDGE('',*,*,#55861,.T.);
#82218=ORIENTED_EDGE('',*,*,#55914,.F.);
#82219=ORIENTED_EDGE('',*,*,#55761,.T.);
#82220=ORIENTED_EDGE('',*,*,#55804,.T.);
#82221=ORIENTED_EDGE('',*,*,#55856,.T.);
#82222=ORIENTED_EDGE('',*,*,#55916,.F.);
#82223=ORIENTED_EDGE('',*,*,#55756,.T.);
#82224=ORIENTED_EDGE('',*,*,#55707,.T.);
#82225=ORIENTED_EDGE('',*,*,#55757,.T.);
#82226=ORIENTED_EDGE('',*,*,#55916,.T.);
#82227=ORIENTED_EDGE('',*,*,#55855,.T.);
#82228=ORIENTED_EDGE('',*,*,#55905,.T.);
#82229=ORIENTED_EDGE('',*,*,#55851,.T.);
#82230=ORIENTED_EDGE('',*,*,#55644,.F.);
#82231=ORIENTED_EDGE('',*,*,#55745,.T.);
#82232=ORIENTED_EDGE('',*,*,#55917,.T.);
#82233=ORIENTED_EDGE('',*,*,#55843,.T.);
#82234=ORIENTED_EDGE('',*,*,#55797,.T.);
#82235=ORIENTED_EDGE('',*,*,#55752,.T.);
#82236=ORIENTED_EDGE('',*,*,#55799,.T.);
#82237=ORIENTED_EDGE('',*,*,#55847,.T.);
#82238=ORIENTED_EDGE('',*,*,#55918,.F.);
#82239=ORIENTED_EDGE('',*,*,#55744,.T.);
#82240=ORIENTED_EDGE('',*,*,#55723,.T.);
#82241=ORIENTED_EDGE('',*,*,#55748,.T.);
#82242=ORIENTED_EDGE('',*,*,#55918,.T.);
#82243=ORIENTED_EDGE('',*,*,#55846,.T.);
#82244=ORIENTED_EDGE('',*,*,#55900,.T.);
#82245=ORIENTED_EDGE('',*,*,#55844,.T.);
#82246=ORIENTED_EDGE('',*,*,#55917,.F.);
#82247=ORIENTED_EDGE('',*,*,#55740,.T.);
#82248=ORIENTED_EDGE('',*,*,#55919,.T.);
#82249=ORIENTED_EDGE('',*,*,#55838,.T.);
#82250=ORIENTED_EDGE('',*,*,#55794,.T.);
#82251=ORIENTED_EDGE('',*,*,#55747,.T.);
#82252=ORIENTED_EDGE('',*,*,#55796,.T.);
#82253=ORIENTED_EDGE('',*,*,#55842,.T.);
#82254=ORIENTED_EDGE('',*,*,#55920,.F.);
#82255=ORIENTED_EDGE('',*,*,#55739,.T.);
#82256=ORIENTED_EDGE('',*,*,#55725,.T.);
#82257=ORIENTED_EDGE('',*,*,#55743,.T.);
#82258=ORIENTED_EDGE('',*,*,#55920,.T.);
#82259=ORIENTED_EDGE('',*,*,#55841,.T.);
#82260=ORIENTED_EDGE('',*,*,#55899,.T.);
#82261=ORIENTED_EDGE('',*,*,#55839,.T.);
#82262=ORIENTED_EDGE('',*,*,#55919,.F.);
#82263=ORIENTED_EDGE('',*,*,#55733,.T.);
#82264=ORIENTED_EDGE('',*,*,#55921,.T.);
#82265=ORIENTED_EDGE('',*,*,#55831,.T.);
#82266=ORIENTED_EDGE('',*,*,#55790,.T.);
#82267=ORIENTED_EDGE('',*,*,#55742,.T.);
#82268=ORIENTED_EDGE('',*,*,#55793,.T.);
#82269=ORIENTED_EDGE('',*,*,#55837,.T.);
#82270=ORIENTED_EDGE('',*,*,#55922,.F.);
#82271=ORIENTED_EDGE('',*,*,#55737,.T.);
#82272=ORIENTED_EDGE('',*,*,#55703,.T.);
#82273=ORIENTED_EDGE('',*,*,#55738,.T.);
#82274=ORIENTED_EDGE('',*,*,#55922,.T.);
#82275=ORIENTED_EDGE('',*,*,#55836,.T.);
#82276=ORIENTED_EDGE('',*,*,#55898,.T.);
#82277=ORIENTED_EDGE('',*,*,#55832,.T.);
#82278=ORIENTED_EDGE('',*,*,#55921,.F.);
#82279=ORIENTED_EDGE('',*,*,#55729,.T.);
#82280=ORIENTED_EDGE('',*,*,#55923,.T.);
#82281=ORIENTED_EDGE('',*,*,#55731,.F.);
#82282=ORIENTED_EDGE('',*,*,#55924,.F.);
#82283=ORIENTED_EDGE('',*,*,#55727,.T.);
#82284=ORIENTED_EDGE('',*,*,#55924,.T.);
#82285=ORIENTED_EDGE('',*,*,#55730,.F.);
#82286=ORIENTED_EDGE('',*,*,#55700,.F.);
#82287=ORIENTED_EDGE('',*,*,#55728,.T.);
#82288=ORIENTED_EDGE('',*,*,#55702,.F.);
#82289=ORIENTED_EDGE('',*,*,#55732,.F.);
#82290=ORIENTED_EDGE('',*,*,#55923,.F.);
#82291=ORIENTED_EDGE('',*,*,#55925,.T.);
#82292=ORIENTED_EDGE('',*,*,#55926,.T.);
#82293=ORIENTED_EDGE('',*,*,#55927,.T.);
#82294=ORIENTED_EDGE('',*,*,#55926,.F.);
#82295=ORIENTED_EDGE('',*,*,#55928,.F.);
#82296=ORIENTED_EDGE('',*,*,#55929,.T.);
#82297=ORIENTED_EDGE('',*,*,#55930,.F.);
#82298=ORIENTED_EDGE('',*,*,#55931,.F.);
#82299=ORIENTED_EDGE('',*,*,#55932,.F.);
#82300=ORIENTED_EDGE('',*,*,#55933,.T.);
#82301=ORIENTED_EDGE('',*,*,#55934,.F.);
#82302=ORIENTED_EDGE('',*,*,#55929,.F.);
#82303=ORIENTED_EDGE('',*,*,#55935,.F.);
#82304=ORIENTED_EDGE('',*,*,#55936,.T.);
#82305=ORIENTED_EDGE('',*,*,#55937,.F.);
#82306=ORIENTED_EDGE('',*,*,#55933,.F.);
#82307=ORIENTED_EDGE('',*,*,#55938,.F.);
#82308=ORIENTED_EDGE('',*,*,#55931,.T.);
#82309=ORIENTED_EDGE('',*,*,#55939,.F.);
#82310=ORIENTED_EDGE('',*,*,#55936,.F.);
#82311=ORIENTED_EDGE('',*,*,#55930,.T.);
#82312=ORIENTED_EDGE('',*,*,#55934,.T.);
#82313=ORIENTED_EDGE('',*,*,#55937,.T.);
#82314=ORIENTED_EDGE('',*,*,#55939,.T.);
#82315=ORIENTED_EDGE('',*,*,#55927,.F.);
#82316=ORIENTED_EDGE('',*,*,#55928,.T.);
#82317=ORIENTED_EDGE('',*,*,#55938,.T.);
#82318=ORIENTED_EDGE('',*,*,#55935,.T.);
#82319=ORIENTED_EDGE('',*,*,#55932,.T.);
#82320=ORIENTED_EDGE('',*,*,#55925,.F.);
#87575=CYLINDRICAL_SURFACE('',#103345,32.4);
#87576=CYLINDRICAL_SURFACE('',#103347,23.324544);
#87577=CYLINDRICAL_SURFACE('',#103348,5.77396800000001);
#87578=CYLINDRICAL_SURFACE('',#103351,5.77396800000001);
#87579=CYLINDRICAL_SURFACE('',#103354,5.77396800000001);
#87580=CYLINDRICAL_SURFACE('',#103357,5.77396800000001);
#87581=CYLINDRICAL_SURFACE('',#103360,5.77396800000001);
#87582=CYLINDRICAL_SURFACE('',#103363,5.77396800000001);
#87583=CYLINDRICAL_SURFACE('',#103366,23.324544);
#87584=CYLINDRICAL_SURFACE('',#103367,15.12);
#87585=CYLINDRICAL_SURFACE('',#103424,49.6934108978581);
#87586=CYLINDRICAL_SURFACE('',#103426,49.6934108978581);
#87587=CYLINDRICAL_SURFACE('',#103428,49.6934108978581);
#87588=CYLINDRICAL_SURFACE('',#103430,49.6934108978581);
#87589=CYLINDRICAL_SURFACE('',#103432,49.6934108978581);
#87590=CYLINDRICAL_SURFACE('',#103434,49.6934108978581);
#87591=CYLINDRICAL_SURFACE('',#103436,49.6934108978581);
#87592=CYLINDRICAL_SURFACE('',#103438,49.6934108978581);
#87593=CYLINDRICAL_SURFACE('',#103440,49.6934108978581);
#87594=CYLINDRICAL_SURFACE('',#103442,49.6934108978581);
#87595=CYLINDRICAL_SURFACE('',#103444,49.6934108978581);
#87596=CYLINDRICAL_SURFACE('',#103446,49.6934108978581);
#87597=CYLINDRICAL_SURFACE('',#103448,49.6934108978581);
#87598=CYLINDRICAL_SURFACE('',#103450,49.6934108978581);
#87599=CYLINDRICAL_SURFACE('',#103482,49.6934108978581);
#87600=CYLINDRICAL_SURFACE('',#103496,23.324544);
#87601=CYLINDRICAL_SURFACE('',#103497,23.324544);
#87602=CYLINDRICAL_SURFACE('',#103498,5.77396800000001);
#87603=CYLINDRICAL_SURFACE('',#103499,23.324544);
#87604=CYLINDRICAL_SURFACE('',#103500,5.773968);
#87605=CYLINDRICAL_SURFACE('',#103501,23.324544);
#87606=CYLINDRICAL_SURFACE('',#103502,23.324544);
#87607=CYLINDRICAL_SURFACE('',#103503,23.324544);
#87608=CYLINDRICAL_SURFACE('',#103504,23.324544);
#87609=CYLINDRICAL_SURFACE('',#103505,23.324544);
#87610=CYLINDRICAL_SURFACE('',#103506,23.324544);
#87611=CYLINDRICAL_SURFACE('',#103507,23.324544);
#87612=CYLINDRICAL_SURFACE('',#103508,23.324544);
#87613=CYLINDRICAL_SURFACE('',#103509,23.324544);
#87614=CYLINDRICAL_SURFACE('',#103510,23.324544);
#87615=CYLINDRICAL_SURFACE('',#103511,5.773968);
#87616=CYLINDRICAL_SURFACE('',#103512,23.324544);
#87617=CYLINDRICAL_SURFACE('',#103513,23.324544);
#87618=CYLINDRICAL_SURFACE('',#103514,23.324544);
#87619=CYLINDRICAL_SURFACE('',#103515,23.324544);
#87620=CYLINDRICAL_SURFACE('',#103516,23.324544);
#87621=CYLINDRICAL_SURFACE('',#103517,23.324544);
#87622=CYLINDRICAL_SURFACE('',#103518,5.773968);
#87623=CYLINDRICAL_SURFACE('',#103519,23.324544);
#87624=CYLINDRICAL_SURFACE('',#103520,23.324544);
#87625=CYLINDRICAL_SURFACE('',#103521,5.77396800000001);
#87626=CYLINDRICAL_SURFACE('',#103522,23.324544);
#87627=CYLINDRICAL_SURFACE('',#103523,5.773968);
#87628=CYLINDRICAL_SURFACE('',#103524,23.324544);
#87629=CYLINDRICAL_SURFACE('',#103525,23.324544);
#87630=CYLINDRICAL_SURFACE('',#103526,5.773968);
#87631=CYLINDRICAL_SURFACE('',#103527,23.324544);
#87632=CYLINDRICAL_SURFACE('',#103528,23.324544);
#87633=CYLINDRICAL_SURFACE('',#103529,5.773968);
#87634=CYLINDRICAL_SURFACE('',#103530,23.324544);
#87635=CYLINDRICAL_SURFACE('',#103531,23.324544);
#87636=CYLINDRICAL_SURFACE('',#103532,5.773968);
#87637=CYLINDRICAL_SURFACE('',#103536,10.12);
#87638=CYLINDRICAL_SURFACE('',#103539,15.12);
#92914=ADVANCED_FACE('',(#13635),#4024,.F.);
#92915=ADVANCED_FACE('',(#13636),#87575,.T.);
#92916=ADVANCED_FACE('',(#13637),#87576,.T.);
#92917=ADVANCED_FACE('',(#13638),#87577,.F.);
#92918=ADVANCED_FACE('',(#13639),#87578,.F.);
#92919=ADVANCED_FACE('',(#13640),#87579,.F.);
#92920=ADVANCED_FACE('',(#13641),#87580,.F.);
#92921=ADVANCED_FACE('',(#13642),#87581,.F.);
#92922=ADVANCED_FACE('',(#13643),#87582,.F.);
#92923=ADVANCED_FACE('',(#13644),#87583,.T.);
#92924=ADVANCED_FACE('',(#13645),#87584,.F.);
#92925=ADVANCED_FACE('',(#13646,#7622),#8524,.F.);
#92926=ADVANCED_FACE('',(#13647,#7623),#8525,.T.);
#92927=ADVANCED_FACE('',(#13648),#4025,.T.);
#92928=ADVANCED_FACE('',(#13649),#4026,.T.);
#92929=ADVANCED_FACE('',(#13650),#4027,.T.);
#92930=ADVANCED_FACE('',(#13651),#4028,.T.);
#92931=ADVANCED_FACE('',(#13652),#4029,.T.);
#92932=ADVANCED_FACE('',(#13653),#4030,.T.);
#92933=ADVANCED_FACE('',(#13654),#4031,.T.);
#92934=ADVANCED_FACE('',(#13655),#4032,.T.);
#92935=ADVANCED_FACE('',(#13656),#4033,.T.);
#92936=ADVANCED_FACE('',(#13657),#4034,.T.);
#92937=ADVANCED_FACE('',(#13658),#4035,.T.);
#92938=ADVANCED_FACE('',(#13659),#4036,.T.);
#92939=ADVANCED_FACE('',(#13660),#4037,.T.);
#92940=ADVANCED_FACE('',(#13661),#4038,.T.);
#92941=ADVANCED_FACE('',(#13662),#87585,.T.);
#92942=ADVANCED_FACE('',(#13663),#87586,.T.);
#92943=ADVANCED_FACE('',(#13664),#87587,.T.);
#92944=ADVANCED_FACE('',(#13665),#87588,.T.);
#92945=ADVANCED_FACE('',(#13666),#87589,.T.);
#92946=ADVANCED_FACE('',(#13667),#87590,.T.);
#92947=ADVANCED_FACE('',(#13668),#87591,.T.);
#92948=ADVANCED_FACE('',(#13669),#87592,.T.);
#92949=ADVANCED_FACE('',(#13670),#87593,.T.);
#92950=ADVANCED_FACE('',(#13671),#87594,.T.);
#92951=ADVANCED_FACE('',(#13672),#87595,.T.);
#92952=ADVANCED_FACE('',(#13673),#87596,.T.);
#92953=ADVANCED_FACE('',(#13674),#87597,.T.);
#92954=ADVANCED_FACE('',(#13675),#87598,.T.);
#92955=ADVANCED_FACE('',(#13676),#4039,.T.);
#92956=ADVANCED_FACE('',(#13677),#4040,.T.);
#92957=ADVANCED_FACE('',(#13678),#4041,.T.);
#92958=ADVANCED_FACE('',(#13679),#4042,.T.);
#92959=ADVANCED_FACE('',(#13680),#4043,.T.);
#92960=ADVANCED_FACE('',(#13681),#4044,.T.);
#92961=ADVANCED_FACE('',(#13682),#4045,.T.);
#92962=ADVANCED_FACE('',(#13683),#4046,.T.);
#92963=ADVANCED_FACE('',(#13684),#4047,.T.);
#92964=ADVANCED_FACE('',(#13685),#4048,.T.);
#92965=ADVANCED_FACE('',(#13686),#4049,.T.);
#92966=ADVANCED_FACE('',(#13687),#4050,.T.);
#92967=ADVANCED_FACE('',(#13688),#4051,.T.);
#92968=ADVANCED_FACE('',(#13689),#4052,.T.);
#92969=ADVANCED_FACE('',(#13690),#4053,.T.);
#92970=ADVANCED_FACE('',(#13691),#87599,.T.);
#92971=ADVANCED_FACE('',(#13692),#4054,.T.);
#92972=ADVANCED_FACE('',(#13693,#7624),#8526,.F.);
#92973=ADVANCED_FACE('',(#13694),#87600,.T.);
#92974=ADVANCED_FACE('',(#13695),#87601,.T.);
#92975=ADVANCED_FACE('',(#13696),#87602,.F.);
#92976=ADVANCED_FACE('',(#13697),#87603,.T.);
#92977=ADVANCED_FACE('',(#13698),#87604,.F.);
#92978=ADVANCED_FACE('',(#13699),#87605,.T.);
#92979=ADVANCED_FACE('',(#13700),#87606,.T.);
#92980=ADVANCED_FACE('',(#13701),#87607,.T.);
#92981=ADVANCED_FACE('',(#13702),#87608,.T.);
#92982=ADVANCED_FACE('',(#13703),#87609,.T.);
#92983=ADVANCED_FACE('',(#13704),#87610,.T.);
#92984=ADVANCED_FACE('',(#13705),#87611,.T.);
#92985=ADVANCED_FACE('',(#13706),#87612,.T.);
#92986=ADVANCED_FACE('',(#13707),#87613,.T.);
#92987=ADVANCED_FACE('',(#13708),#87614,.T.);
#92988=ADVANCED_FACE('',(#13709),#87615,.F.);
#92989=ADVANCED_FACE('',(#13710),#87616,.T.);
#92990=ADVANCED_FACE('',(#13711),#87617,.T.);
#92991=ADVANCED_FACE('',(#13712),#87618,.T.);
#92992=ADVANCED_FACE('',(#13713),#87619,.T.);
#92993=ADVANCED_FACE('',(#13714),#87620,.T.);
#92994=ADVANCED_FACE('',(#13715),#87621,.T.);
#92995=ADVANCED_FACE('',(#13716),#87622,.F.);
#92996=ADVANCED_FACE('',(#13717),#87623,.T.);
#92997=ADVANCED_FACE('',(#13718),#87624,.T.);
#92998=ADVANCED_FACE('',(#13719),#87625,.F.);
#92999=ADVANCED_FACE('',(#13720),#87626,.T.);
#93000=ADVANCED_FACE('',(#13721),#87627,.F.);
#93001=ADVANCED_FACE('',(#13722),#87628,.T.);
#93002=ADVANCED_FACE('',(#13723),#87629,.T.);
#93003=ADVANCED_FACE('',(#13724),#87630,.F.);
#93004=ADVANCED_FACE('',(#13725),#87631,.T.);
#93005=ADVANCED_FACE('',(#13726),#87632,.T.);
#93006=ADVANCED_FACE('',(#13727),#87633,.F.);
#93007=ADVANCED_FACE('',(#13728),#87634,.T.);
#93008=ADVANCED_FACE('',(#13729),#87635,.T.);
#93009=ADVANCED_FACE('',(#13730),#87636,.F.);
#93010=ADVANCED_FACE('',(#13731),#8527,.T.);
#93011=ADVANCED_FACE('',(#13732),#8528,.T.);
#93012=ADVANCED_FACE('',(#13733),#8529,.T.);
#93013=ADVANCED_FACE('',(#13734),#87637,.F.);
#93014=ADVANCED_FACE('',(#13735),#87638,.T.);
#93015=ADVANCED_FACE('',(#13736),#8530,.T.);
#93016=ADVANCED_FACE('',(#13737),#8531,.T.);
#93017=ADVANCED_FACE('',(#13738),#8532,.T.);
#93018=ADVANCED_FACE('',(#13739,#7625),#8533,.T.);
#93019=ADVANCED_FACE('',(#13740,#7626),#8534,.F.);
#93729=CLOSED_SHELL('',(#92914,#92915,#92916,#92917,#92918,#92919,#92920,
#92921,#92922,#92923,#92924,#92925,#92926,#92927,#92928,#92929,#92930,#92931,
#92932,#92933,#92934,#92935,#92936,#92937,#92938,#92939,#92940,#92941,#92942,
#92943,#92944,#92945,#92946,#92947,#92948,#92949,#92950,#92951,#92952,#92953,
#92954,#92955,#92956,#92957,#92958,#92959,#92960,#92961,#92962,#92963,#92964,
#92965,#92966,#92967,#92968,#92969,#92970,#92971,#92972,#92973,#92974,#92975,
#92976,#92977,#92978,#92979,#92980,#92981,#92982,#92983,#92984,#92985,#92986,
#92987,#92988,#92989,#92990,#92991,#92992,#92993,#92994,#92995,#92996,#92997,
#92998,#92999,#93000,#93001,#93002,#93003,#93004,#93005,#93006,#93007,#93008,
#93009,#93010,#93011,#93012));
#93730=CLOSED_SHELL('',(#93013,#93014,#93015,#93016,#93017,#93018,#93019));
#103340=AXIS2_PLACEMENT_3D('',#271223,#127341,#127342);
#103341=AXIS2_PLACEMENT_3D('',#271224,#127343,#127344);
#103342=AXIS2_PLACEMENT_3D('',#271226,#127345,#127346);
#103343=AXIS2_PLACEMENT_3D('',#271228,#127347,#127348);
#103344=AXIS2_PLACEMENT_3D('',#271229,#127349,#127350);
#103345=AXIS2_PLACEMENT_3D('',#271230,#127351,#127352);
#103346=AXIS2_PLACEMENT_3D('',#271233,#127354,#127355);
#103347=AXIS2_PLACEMENT_3D('',#271234,#127356,#127357);
#103348=AXIS2_PLACEMENT_3D('',#271255,#127360,#127361);
#103349=AXIS2_PLACEMENT_3D('',#271272,#127363,#127364);
#103350=AXIS2_PLACEMENT_3D('',#271289,#127366,#127367);
#103351=AXIS2_PLACEMENT_3D('',#271290,#127368,#127369);
#103352=AXIS2_PLACEMENT_3D('',#271293,#127370,#127371);
#103353=AXIS2_PLACEMENT_3D('',#271309,#127373,#127374);
#103354=AXIS2_PLACEMENT_3D('',#271325,#127376,#127377);
#103355=AXIS2_PLACEMENT_3D('',#271328,#127378,#127379);
#103356=AXIS2_PLACEMENT_3D('',#271344,#127381,#127382);
#103357=AXIS2_PLACEMENT_3D('',#271360,#127384,#127385);
#103358=AXIS2_PLACEMENT_3D('',#271370,#127386,#127387);
#103359=AXIS2_PLACEMENT_3D('',#271386,#127389,#127390);
#103360=AXIS2_PLACEMENT_3D('',#271395,#127392,#127393);
#103361=AXIS2_PLACEMENT_3D('',#271398,#127394,#127395);
#103362=AXIS2_PLACEMENT_3D('',#271414,#127397,#127398);
#103363=AXIS2_PLACEMENT_3D('',#271430,#127400,#127401);
#103364=AXIS2_PLACEMENT_3D('',#271433,#127402,#127403);
#103365=AXIS2_PLACEMENT_3D('',#271449,#127405,#127406);
#103366=AXIS2_PLACEMENT_3D('',#271465,#127408,#127409);
#103367=AXIS2_PLACEMENT_3D('',#271486,#127412,#127413);
#103368=AXIS2_PLACEMENT_3D('',#271489,#127414,#127415);
#103369=AXIS2_PLACEMENT_3D('',#271493,#127417,#127418);
#103370=AXIS2_PLACEMENT_3D('',#271495,#127420,#127421);
#103371=AXIS2_PLACEMENT_3D('',#271498,#127422,#127423);
#103372=AXIS2_PLACEMENT_3D('',#271500,#127424,#127425);
#103373=AXIS2_PLACEMENT_3D('',#271502,#127426,#127427);
#103374=AXIS2_PLACEMENT_3D('',#271504,#127428,#127429);
#103375=AXIS2_PLACEMENT_3D('',#271506,#127430,#127431);
#103376=AXIS2_PLACEMENT_3D('',#271508,#127432,#127433);
#103377=AXIS2_PLACEMENT_3D('',#271510,#127434,#127435);
#103378=AXIS2_PLACEMENT_3D('',#271512,#127436,#127437);
#103379=AXIS2_PLACEMENT_3D('',#271514,#127438,#127439);
#103380=AXIS2_PLACEMENT_3D('',#271515,#127440,#127441);
#103381=AXIS2_PLACEMENT_3D('',#271516,#127442,#127443);
#103382=AXIS2_PLACEMENT_3D('',#271517,#127444,#127445);
#103383=AXIS2_PLACEMENT_3D('',#271518,#127446,#127447);
#103384=AXIS2_PLACEMENT_3D('',#271519,#127448,#127449);
#103385=AXIS2_PLACEMENT_3D('',#271520,#127450,#127451);
#103386=AXIS2_PLACEMENT_3D('',#271522,#127452,#127453);
#103387=AXIS2_PLACEMENT_3D('',#271524,#127454,#127455);
#103388=AXIS2_PLACEMENT_3D('',#271526,#127456,#127457);
#103389=AXIS2_PLACEMENT_3D('',#271528,#127458,#127459);
#103390=AXIS2_PLACEMENT_3D('',#271530,#127460,#127461);
#103391=AXIS2_PLACEMENT_3D('',#271532,#127462,#127463);
#103392=AXIS2_PLACEMENT_3D('',#271534,#127464,#127465);
#103393=AXIS2_PLACEMENT_3D('',#271536,#127466,#127467);
#103394=AXIS2_PLACEMENT_3D('',#271537,#127468,#127469);
#103395=AXIS2_PLACEMENT_3D('',#271543,#127473,#127474);
#103396=AXIS2_PLACEMENT_3D('',#271549,#127478,#127479);
#103397=AXIS2_PLACEMENT_3D('',#271561,#127480,#127481);
#103398=AXIS2_PLACEMENT_3D('',#271581,#127482,#127483);
#103399=AXIS2_PLACEMENT_3D('',#271606,#127484,#127485);
#103400=AXIS2_PLACEMENT_3D('',#271613,#127486,#127487);
#103401=AXIS2_PLACEMENT_3D('',#271638,#127488,#127489);
#103402=AXIS2_PLACEMENT_3D('',#271645,#127490,#127491);
#103403=AXIS2_PLACEMENT_3D('',#271670,#127492,#127493);
#103404=AXIS2_PLACEMENT_3D('',#271677,#127494,#127495);
#103405=AXIS2_PLACEMENT_3D('',#271679,#127496,#127497);
#103406=AXIS2_PLACEMENT_3D('',#271699,#127498,#127499);
#103407=AXIS2_PLACEMENT_3D('',#271724,#127500,#127501);
#103408=AXIS2_PLACEMENT_3D('',#271731,#127502,#127503);
#103409=AXIS2_PLACEMENT_3D('',#271743,#127504,#127505);
#103410=AXIS2_PLACEMENT_3D('',#271763,#127506,#127507);
#103411=AXIS2_PLACEMENT_3D('',#271774,#127508,#127509);
#103412=AXIS2_PLACEMENT_3D('',#271781,#127510,#127511);
#103413=AXIS2_PLACEMENT_3D('',#271799,#127512,#127513);
#103414=AXIS2_PLACEMENT_3D('',#271806,#127514,#127515);
#103415=AXIS2_PLACEMENT_3D('',#271817,#127516,#127517);
#103416=AXIS2_PLACEMENT_3D('',#271824,#127518,#127519);
#103417=AXIS2_PLACEMENT_3D('',#271835,#127520,#127521);
#103418=AXIS2_PLACEMENT_3D('',#271842,#127522,#127523);
#103419=AXIS2_PLACEMENT_3D('',#271853,#127524,#127525);
#103420=AXIS2_PLACEMENT_3D('',#271860,#127526,#127527);
#103421=AXIS2_PLACEMENT_3D('',#271871,#127528,#127529);
#103422=AXIS2_PLACEMENT_3D('',#271885,#127530,#127531);
#103423=AXIS2_PLACEMENT_3D('',#271896,#127532,#127533);
#103424=AXIS2_PLACEMENT_3D('',#271903,#127534,#127535);
#103425=AXIS2_PLACEMENT_3D('',#271907,#127537,#127538);
#103426=AXIS2_PLACEMENT_3D('',#271909,#127540,#127541);
#103427=AXIS2_PLACEMENT_3D('',#271914,#127544,#127545);
#103428=AXIS2_PLACEMENT_3D('',#271915,#127546,#127547);
#103429=AXIS2_PLACEMENT_3D('',#271920,#127550,#127551);
#103430=AXIS2_PLACEMENT_3D('',#271921,#127552,#127553);
#103431=AXIS2_PLACEMENT_3D('',#271926,#127556,#127557);
#103432=AXIS2_PLACEMENT_3D('',#271927,#127558,#127559);
#103433=AXIS2_PLACEMENT_3D('',#271929,#127560,#127561);
#103434=AXIS2_PLACEMENT_3D('',#271931,#127563,#127564);
#103435=AXIS2_PLACEMENT_3D('',#271936,#127567,#127568);
#103436=AXIS2_PLACEMENT_3D('',#271937,#127569,#127570);
#103437=AXIS2_PLACEMENT_3D('',#271941,#127572,#127573);
#103438=AXIS2_PLACEMENT_3D('',#271943,#127575,#127576);
#103439=AXIS2_PLACEMENT_3D('',#271947,#127578,#127579);
#103440=AXIS2_PLACEMENT_3D('',#271949,#127581,#127582);
#103441=AXIS2_PLACEMENT_3D('',#271954,#127585,#127586);
#103442=AXIS2_PLACEMENT_3D('',#271955,#127587,#127588);
#103443=AXIS2_PLACEMENT_3D('',#271959,#127590,#127591);
#103444=AXIS2_PLACEMENT_3D('',#271961,#127593,#127594);
#103445=AXIS2_PLACEMENT_3D('',#271965,#127596,#127597);
#103446=AXIS2_PLACEMENT_3D('',#271967,#127599,#127600);
#103447=AXIS2_PLACEMENT_3D('',#271972,#127603,#127604);
#103448=AXIS2_PLACEMENT_3D('',#271973,#127605,#127606);
#103449=AXIS2_PLACEMENT_3D('',#271977,#127608,#127609);
#103450=AXIS2_PLACEMENT_3D('',#271979,#127611,#127612);
#103451=AXIS2_PLACEMENT_3D('',#271984,#127615,#127616);
#103452=AXIS2_PLACEMENT_3D('',#271985,#127617,#127618);
#103453=AXIS2_PLACEMENT_3D('',#272001,#127619,#127620);
#103454=AXIS2_PLACEMENT_3D('',#272015,#127621,#127622);
#103455=AXIS2_PLACEMENT_3D('',#272044,#127623,#127624);
#103456=AXIS2_PLACEMENT_3D('',#272045,#127625,#127626);
#103457=AXIS2_PLACEMENT_3D('',#272074,#127627,#127628);
#103458=AXIS2_PLACEMENT_3D('',#272075,#127629,#127630);
#103459=AXIS2_PLACEMENT_3D('',#272104,#127631,#127632);
#103460=AXIS2_PLACEMENT_3D('',#272105,#127633,#127634);
#103461=AXIS2_PLACEMENT_3D('',#272114,#127635,#127636);
#103462=AXIS2_PLACEMENT_3D('',#272128,#127637,#127638);
#103463=AXIS2_PLACEMENT_3D('',#272157,#127639,#127640);
#103464=AXIS2_PLACEMENT_3D('',#272158,#127641,#127642);
#103465=AXIS2_PLACEMENT_3D('',#272174,#127643,#127644);
#103466=AXIS2_PLACEMENT_3D('',#272188,#127645,#127646);
#103467=AXIS2_PLACEMENT_3D('',#272195,#127647,#127648);
#103468=AXIS2_PLACEMENT_3D('',#272204,#127649,#127650);
#103469=AXIS2_PLACEMENT_3D('',#272227,#127651,#127652);
#103470=AXIS2_PLACEMENT_3D('',#272228,#127653,#127654);
#103471=AXIS2_PLACEMENT_3D('',#272235,#127655,#127656);
#103472=AXIS2_PLACEMENT_3D('',#272244,#127657,#127658);
#103473=AXIS2_PLACEMENT_3D('',#272251,#127659,#127660);
#103474=AXIS2_PLACEMENT_3D('',#272260,#127661,#127662);
#103475=AXIS2_PLACEMENT_3D('',#272275,#127663,#127664);
#103476=AXIS2_PLACEMENT_3D('',#272276,#127665,#127666);
#103477=AXIS2_PLACEMENT_3D('',#272284,#127667,#127668);
#103478=AXIS2_PLACEMENT_3D('',#272298,#127669,#127670);
#103479=AXIS2_PLACEMENT_3D('',#272313,#127671,#127672);
#103480=AXIS2_PLACEMENT_3D('',#272314,#127673,#127674);
#103481=AXIS2_PLACEMENT_3D('',#272337,#127675,#127676);
#103482=AXIS2_PLACEMENT_3D('',#272338,#127677,#127678);
#103483=AXIS2_PLACEMENT_3D('',#272341,#127680,#127681);
#103484=AXIS2_PLACEMENT_3D('',#272342,#127682,#127683);
#103485=AXIS2_PLACEMENT_3D('',#272362,#127684,#127685);
#103486=AXIS2_PLACEMENT_3D('',#272363,#127686,#127687);
#103487=AXIS2_PLACEMENT_3D('',#272364,#127688,#127689);
#103488=AXIS2_PLACEMENT_3D('',#272365,#127690,#127691);
#103489=AXIS2_PLACEMENT_3D('',#272366,#127692,#127693);
#103490=AXIS2_PLACEMENT_3D('',#272367,#127694,#127695);
#103491=AXIS2_PLACEMENT_3D('',#272368,#127696,#127697);
#103492=AXIS2_PLACEMENT_3D('',#272369,#127698,#127699);
#103493=AXIS2_PLACEMENT_3D('',#272370,#127700,#127701);
#103494=AXIS2_PLACEMENT_3D('',#272371,#127702,#127703);
#103495=AXIS2_PLACEMENT_3D('',#272372,#127704,#127705);
#103496=AXIS2_PLACEMENT_3D('',#272373,#127706,#127707);
#103497=AXIS2_PLACEMENT_3D('',#272375,#127709,#127710);
#103498=AXIS2_PLACEMENT_3D('',#272377,#127712,#127713);
#103499=AXIS2_PLACEMENT_3D('',#272378,#127714,#127715);
#103500=AXIS2_PLACEMENT_3D('',#272380,#127717,#127718);
#103501=AXIS2_PLACEMENT_3D('',#272381,#127719,#127720);
#103502=AXIS2_PLACEMENT_3D('',#272382,#127721,#127722);
#103503=AXIS2_PLACEMENT_3D('',#272383,#127723,#127724);
#103504=AXIS2_PLACEMENT_3D('',#272384,#127725,#127726);
#103505=AXIS2_PLACEMENT_3D('',#272385,#127727,#127728);
#103506=AXIS2_PLACEMENT_3D('',#272386,#127729,#127730);
#103507=AXIS2_PLACEMENT_3D('',#272387,#127731,#127732);
#103508=AXIS2_PLACEMENT_3D('',#272388,#127733,#127734);
#103509=AXIS2_PLACEMENT_3D('',#272389,#127735,#127736);
#103510=AXIS2_PLACEMENT_3D('',#272391,#127738,#127739);
#103511=AXIS2_PLACEMENT_3D('',#272393,#127741,#127742);
#103512=AXIS2_PLACEMENT_3D('',#272394,#127743,#127744);
#103513=AXIS2_PLACEMENT_3D('',#272395,#127745,#127746);
#103514=AXIS2_PLACEMENT_3D('',#272396,#127747,#127748);
#103515=AXIS2_PLACEMENT_3D('',#272397,#127749,#127750);
#103516=AXIS2_PLACEMENT_3D('',#272398,#127751,#127752);
#103517=AXIS2_PLACEMENT_3D('',#272400,#127754,#127755);
#103518=AXIS2_PLACEMENT_3D('',#272402,#127757,#127758);
#103519=AXIS2_PLACEMENT_3D('',#272403,#127759,#127760);
#103520=AXIS2_PLACEMENT_3D('',#272405,#127762,#127763);
#103521=AXIS2_PLACEMENT_3D('',#272407,#127765,#127766);
#103522=AXIS2_PLACEMENT_3D('',#272408,#127767,#127768);
#103523=AXIS2_PLACEMENT_3D('',#272410,#127770,#127771);
#103524=AXIS2_PLACEMENT_3D('',#272411,#127772,#127773);
#103525=AXIS2_PLACEMENT_3D('',#272413,#127775,#127776);
#103526=AXIS2_PLACEMENT_3D('',#272415,#127778,#127779);
#103527=AXIS2_PLACEMENT_3D('',#272416,#127780,#127781);
#103528=AXIS2_PLACEMENT_3D('',#272418,#127783,#127784);
#103529=AXIS2_PLACEMENT_3D('',#272420,#127786,#127787);
#103530=AXIS2_PLACEMENT_3D('',#272421,#127788,#127789);
#103531=AXIS2_PLACEMENT_3D('',#272423,#127791,#127792);
#103532=AXIS2_PLACEMENT_3D('',#272425,#127794,#127795);
#103533=AXIS2_PLACEMENT_3D('',#272426,#127796,#127797);
#103534=AXIS2_PLACEMENT_3D('',#272429,#127800,#127801);
#103535=AXIS2_PLACEMENT_3D('',#272430,#127802,#127803);
#103536=AXIS2_PLACEMENT_3D('',#272431,#127804,#127805);
#103537=AXIS2_PLACEMENT_3D('',#272433,#127806,#127807);
#103538=AXIS2_PLACEMENT_3D('',#272436,#127809,#127810);
#103539=AXIS2_PLACEMENT_3D('',#272437,#127811,#127812);
#103540=AXIS2_PLACEMENT_3D('',#272440,#127813,#127814);
#103541=AXIS2_PLACEMENT_3D('',#272444,#127816,#127817);
#103542=AXIS2_PLACEMENT_3D('',#272446,#127819,#127820);
#103543=AXIS2_PLACEMENT_3D('',#272452,#127824,#127825);
#103544=AXIS2_PLACEMENT_3D('',#272458,#127829,#127830);
#103545=AXIS2_PLACEMENT_3D('',#272461,#127833,#127834);
#103546=AXIS2_PLACEMENT_3D('',#272462,#127835,#127836);
#127341=DIRECTION('axis',(0.,0.,1.));
#127342=DIRECTION('refdir',(1.,0.,0.));
#127343=DIRECTION('center_axis',(1.,0.,0.));
#127344=DIRECTION('ref_axis',(0.,0.,-1.));
#127345=DIRECTION('center_axis',(1.,0.,0.));
#127346=DIRECTION('ref_axis',(0.,0.,-1.));
#127347=DIRECTION('center_axis',(0.,1.,1.15813679845853E-16));
#127348=DIRECTION('ref_axis',(0.,-1.15813679845853E-16,1.));
#127349=DIRECTION('center_axis',(-1.,0.,0.));
#127350=DIRECTION('ref_axis',(0.,0.,-1.));
#127351=DIRECTION('center_axis',(1.,0.,0.));
#127352=DIRECTION('ref_axis',(0.,0.,-1.));
#127353=DIRECTION('',(-1.,0.,0.));
#127354=DIRECTION('center_axis',(-1.,0.,0.));
#127355=DIRECTION('ref_axis',(0.,0.,1.));
#127356=DIRECTION('center_axis',(-1.,0.,0.));
#127357=DIRECTION('ref_axis',(0.,0.,1.));
#127358=DIRECTION('',(-1.,0.,0.));
#127359=DIRECTION('',(1.,0.,0.));
#127360=DIRECTION('center_axis',(-1.,0.,0.));
#127361=DIRECTION('ref_axis',(0.,0.,1.));
#127362=DIRECTION('',(-1.,0.,0.));
#127363=DIRECTION('center_axis',(-1.,0.,0.));
#127364=DIRECTION('ref_axis',(0.,0.,-1.));
#127365=DIRECTION('',(-1.,0.,0.));
#127366=DIRECTION('center_axis',(1.,0.,0.));
#127367=DIRECTION('ref_axis',(0.,0.587785252292479,-0.809016994374943));
#127368=DIRECTION('center_axis',(-1.,0.,0.));
#127369=DIRECTION('ref_axis',(0.,0.,1.));
#127370=DIRECTION('center_axis',(1.,0.,0.));
#127371=DIRECTION('ref_axis',(0.,0.866025403784443,-0.499999999999992));
#127372=DIRECTION('',(-1.,0.,0.));
#127373=DIRECTION('center_axis',(-1.,0.,0.));
#127374=DIRECTION('ref_axis',(0.,6.00877412544304E-16,-1.));
#127375=DIRECTION('',(-1.,0.,0.));
#127376=DIRECTION('center_axis',(-1.,0.,0.));
#127377=DIRECTION('ref_axis',(0.,0.,1.));
#127378=DIRECTION('center_axis',(1.,0.,0.));
#127379=DIRECTION('ref_axis',(0.,0.743144825477386,0.669130606358867));
#127380=DIRECTION('',(-1.,0.,0.));
#127381=DIRECTION('center_axis',(-1.,0.,0.));
#127382=DIRECTION('ref_axis',(0.,0.,-1.));
#127383=DIRECTION('',(-1.,0.,0.));
#127384=DIRECTION('center_axis',(-1.,0.,0.));
#127385=DIRECTION('ref_axis',(0.,0.,1.));
#127386=DIRECTION('center_axis',(1.,0.,0.));
#127387=DIRECTION('ref_axis',(0.,0.406736643075789,0.913545457642606));
#127388=DIRECTION('',(-1.,0.,0.));
#127389=DIRECTION('center_axis',(-1.,0.,0.));
#127390=DIRECTION('ref_axis',(0.,0.,-1.));
#127391=DIRECTION('',(-1.,0.,0.));
#127392=DIRECTION('center_axis',(-1.,0.,0.));
#127393=DIRECTION('ref_axis',(0.,0.,1.));
#127394=DIRECTION('center_axis',(1.,0.,0.));
#127395=DIRECTION('ref_axis',(0.,0.95105651629515,0.309016994374958));
#127396=DIRECTION('',(-1.,0.,0.));
#127397=DIRECTION('center_axis',(-1.,0.,0.));
#127398=DIRECTION('ref_axis',(0.,-1.80263223763291E-15,-1.));
#127399=DIRECTION('',(-1.,0.,0.));
#127400=DIRECTION('center_axis',(-1.,0.,0.));
#127401=DIRECTION('ref_axis',(0.,0.,1.));
#127402=DIRECTION('center_axis',(1.,0.,0.));
#127403=DIRECTION('ref_axis',(0.,0.994521895368274,-0.104528463267644));
#127404=DIRECTION('',(-1.,0.,0.));
#127405=DIRECTION('center_axis',(-1.,0.,0.));
#127406=DIRECTION('ref_axis',(0.,-2.66639351816535E-15,-1.));
#127407=DIRECTION('',(-1.,0.,0.));
#127408=DIRECTION('center_axis',(-1.,0.,0.));
#127409=DIRECTION('ref_axis',(0.,0.,1.));
#127410=DIRECTION('',(-1.,0.,0.));
#127411=DIRECTION('',(-1.,0.,0.));
#127412=DIRECTION('center_axis',(-1.,0.,0.));
#127413=DIRECTION('ref_axis',(0.,-1.,-1.83697019872103E-16));
#127414=DIRECTION('center_axis',(1.,0.,0.));
#127415=DIRECTION('ref_axis',(0.,0.,1.));
#127416=DIRECTION('',(-1.,0.,0.));
#127417=DIRECTION('center_axis',(1.,0.,0.));
#127418=DIRECTION('ref_axis',(0.,0.,1.));
#127419=DIRECTION('',(1.,0.,0.));
#127420=DIRECTION('center_axis',(-1.,0.,0.));
#127421=DIRECTION('ref_axis',(0.,0.,1.));
#127422=DIRECTION('center_axis',(1.,0.,0.));
#127423=DIRECTION('ref_axis',(0.,-0.994521895368273,-0.104528463267657));
#127424=DIRECTION('center_axis',(-1.,0.,0.));
#127425=DIRECTION('ref_axis',(0.,0.,1.));
#127426=DIRECTION('center_axis',(1.,0.,0.));
#127427=DIRECTION('ref_axis',(0.,-0.866025403784436,-0.500000000000004));
#127428=DIRECTION('center_axis',(-1.,0.,0.));
#127429=DIRECTION('ref_axis',(0.,0.,1.));
#127430=DIRECTION('center_axis',(1.,0.,0.));
#127431=DIRECTION('ref_axis',(0.,-0.587785252292469,-0.80901699437495));
#127432=DIRECTION('center_axis',(-1.,0.,0.));
#127433=DIRECTION('ref_axis',(0.,0.,1.));
#127434=DIRECTION('center_axis',(1.,0.,0.));
#127435=DIRECTION('ref_axis',(0.,-0.207911690817753,-0.978147600733807));
#127436=DIRECTION('center_axis',(-1.,0.,0.));
#127437=DIRECTION('ref_axis',(0.,0.,1.));
#127438=DIRECTION('center_axis',(1.,0.,0.));
#127439=DIRECTION('ref_axis',(0.,0.207911690817766,-0.978147600733804));
#127440=DIRECTION('center_axis',(-1.,0.,0.));
#127441=DIRECTION('ref_axis',(0.,0.,1.));
#127442=DIRECTION('center_axis',(-1.,0.,0.));
#127443=DIRECTION('ref_axis',(0.,0.,1.));
#127444=DIRECTION('center_axis',(-1.,0.,0.));
#127445=DIRECTION('ref_axis',(0.,0.,1.));
#127446=DIRECTION('center_axis',(-1.,0.,0.));
#127447=DIRECTION('ref_axis',(0.,0.,1.));
#127448=DIRECTION('center_axis',(-1.,0.,0.));
#127449=DIRECTION('ref_axis',(0.,0.,1.));
#127450=DIRECTION('center_axis',(-1.,0.,0.));
#127451=DIRECTION('ref_axis',(0.,0.,1.));
#127452=DIRECTION('center_axis',(-1.,0.,0.));
#127453=DIRECTION('ref_axis',(0.,0.,1.));
#127454=DIRECTION('center_axis',(1.,0.,0.));
#127455=DIRECTION('ref_axis',(0.,0.,1.));
#127456=DIRECTION('center_axis',(-1.,0.,0.));
#127457=DIRECTION('ref_axis',(0.,0.,1.));
#127458=DIRECTION('center_axis',(1.,0.,0.));
#127459=DIRECTION('ref_axis',(0.,-0.406736643075801,0.913545457642601));
#127460=DIRECTION('center_axis',(-1.,0.,0.));
#127461=DIRECTION('ref_axis',(0.,0.,1.));
#127462=DIRECTION('center_axis',(1.,0.,0.));
#127463=DIRECTION('ref_axis',(0.,-0.743144825477396,0.669130606358857));
#127464=DIRECTION('center_axis',(-1.,0.,0.));
#127465=DIRECTION('ref_axis',(0.,0.,1.));
#127466=DIRECTION('center_axis',(1.,0.,0.));
#127467=DIRECTION('ref_axis',(0.,-0.951056516295155,0.309016994374945));
#127468=DIRECTION('center_axis',(-1.,0.,0.));
#127469=DIRECTION('ref_axis',(0.,0.,1.));
#127470=DIRECTION('',(0.,1.,0.));
#127471=DIRECTION('',(0.,-1.,0.));
#127472=DIRECTION('',(0.,0.,1.));
#127473=DIRECTION('center_axis',(-1.,0.,0.));
#127474=DIRECTION('ref_axis',(0.,0.,1.));
#127475=DIRECTION('',(0.,1.,0.));
#127476=DIRECTION('',(0.,0.,1.));
#127477=DIRECTION('',(0.,-1.,0.));
#127478=DIRECTION('center_axis',(-1.,0.,0.));
#127479=DIRECTION('ref_axis',(0.,0.,1.));
#127480=DIRECTION('center_axis',(-1.,0.,0.));
#127481=DIRECTION('ref_axis',(0.,0.,1.));
#127482=DIRECTION('center_axis',(-1.,0.,0.));
#127483=DIRECTION('ref_axis',(0.,0.,1.));
#127484=DIRECTION('center_axis',(-1.,0.,0.));
#127485=DIRECTION('ref_axis',(0.,0.,1.));
#127486=DIRECTION('center_axis',(-1.,0.,0.));
#127487=DIRECTION('ref_axis',(0.,0.,1.));
#127488=DIRECTION('center_axis',(-1.,0.,0.));
#127489=DIRECTION('ref_axis',(0.,0.,1.));
#127490=DIRECTION('center_axis',(-1.,0.,0.));
#127491=DIRECTION('ref_axis',(0.,0.,1.));
#127492=DIRECTION('center_axis',(-1.,0.,0.));
#127493=DIRECTION('ref_axis',(0.,0.,1.));
#127494=DIRECTION('center_axis',(-1.,0.,0.));
#127495=DIRECTION('ref_axis',(0.,0.,1.));
#127496=DIRECTION('center_axis',(-1.,0.,0.));
#127497=DIRECTION('ref_axis',(0.,0.,1.));
#127498=DIRECTION('center_axis',(-1.,0.,0.));
#127499=DIRECTION('ref_axis',(0.,0.,1.));
#127500=DIRECTION('center_axis',(-1.,0.,0.));
#127501=DIRECTION('ref_axis',(0.,0.,1.));
#127502=DIRECTION('center_axis',(-1.,0.,0.));
#127503=DIRECTION('ref_axis',(0.,0.,1.));
#127504=DIRECTION('center_axis',(-1.,0.,0.));
#127505=DIRECTION('ref_axis',(0.,0.,1.));
#127506=DIRECTION('center_axis',(-1.,0.,0.));
#127507=DIRECTION('ref_axis',(0.,0.,1.));
#127508=DIRECTION('center_axis',(-1.,0.,0.));
#127509=DIRECTION('ref_axis',(0.,0.,1.));
#127510=DIRECTION('center_axis',(-1.,0.,0.));
#127511=DIRECTION('ref_axis',(0.,0.,1.));
#127512=DIRECTION('center_axis',(-1.,0.,0.));
#127513=DIRECTION('ref_axis',(0.,0.,1.));
#127514=DIRECTION('center_axis',(-1.,0.,0.));
#127515=DIRECTION('ref_axis',(0.,0.,1.));
#127516=DIRECTION('center_axis',(-1.,0.,0.));
#127517=DIRECTION('ref_axis',(0.,0.,1.));
#127518=DIRECTION('center_axis',(-1.,0.,0.));
#127519=DIRECTION('ref_axis',(0.,0.,1.));
#127520=DIRECTION('center_axis',(-1.,0.,0.));
#127521=DIRECTION('ref_axis',(0.,0.,1.));
#127522=DIRECTION('center_axis',(-1.,0.,0.));
#127523=DIRECTION('ref_axis',(0.,0.,1.));
#127524=DIRECTION('center_axis',(-1.,0.,0.));
#127525=DIRECTION('ref_axis',(0.,0.,1.));
#127526=DIRECTION('center_axis',(-1.,0.,0.));
#127527=DIRECTION('ref_axis',(0.,0.,1.));
#127528=DIRECTION('center_axis',(-1.,0.,0.));
#127529=DIRECTION('ref_axis',(0.,0.,1.));
#127530=DIRECTION('center_axis',(-1.,0.,0.));
#127531=DIRECTION('ref_axis',(0.,0.,1.));
#127532=DIRECTION('center_axis',(-1.,0.,0.));
#127533=DIRECTION('ref_axis',(0.,0.,1.));
#127534=DIRECTION('center_axis',(-1.,0.,0.));
#127535=DIRECTION('ref_axis',(0.,0.,1.));
#127536=DIRECTION('',(1.,0.,0.));
#127537=DIRECTION('center_axis',(-1.,0.,0.));
#127538=DIRECTION('ref_axis',(0.,0.,1.));
#127539=DIRECTION('',(-1.,0.,0.));
#127540=DIRECTION('center_axis',(-1.,0.,0.));
#127541=DIRECTION('ref_axis',(0.,0.,1.));
#127542=DIRECTION('',(-1.,0.,0.));
#127543=DIRECTION('',(1.,0.,0.));
#127544=DIRECTION('center_axis',(-1.,0.,0.));
#127545=DIRECTION('ref_axis',(0.,0.,1.));
#127546=DIRECTION('center_axis',(-1.,0.,0.));
#127547=DIRECTION('ref_axis',(0.,0.,1.));
#127548=DIRECTION('',(-1.,0.,0.));
#127549=DIRECTION('',(1.,0.,0.));
#127550=DIRECTION('center_axis',(-1.,0.,0.));
#127551=DIRECTION('ref_axis',(0.,0.,1.));
#127552=DIRECTION('center_axis',(-1.,0.,0.));
#127553=DIRECTION('ref_axis',(0.,0.,1.));
#127554=DIRECTION('',(-1.,0.,0.));
#127555=DIRECTION('',(1.,0.,0.));
#127556=DIRECTION('center_axis',(-1.,0.,0.));
#127557=DIRECTION('ref_axis',(0.,0.,1.));
#127558=DIRECTION('center_axis',(-1.,0.,0.));
#127559=DIRECTION('ref_axis',(0.,0.,1.));
#127560=DIRECTION('center_axis',(-1.,0.,0.));
#127561=DIRECTION('ref_axis',(0.,0.,1.));
#127562=DIRECTION('',(-1.,0.,0.));
#127563=DIRECTION('center_axis',(-1.,0.,0.));
#127564=DIRECTION('ref_axis',(0.,0.,1.));
#127565=DIRECTION('',(-1.,0.,0.));
#127566=DIRECTION('',(1.,0.,0.));
#127567=DIRECTION('center_axis',(-1.,0.,0.));
#127568=DIRECTION('ref_axis',(0.,0.,1.));
#127569=DIRECTION('center_axis',(-1.,0.,0.));
#127570=DIRECTION('ref_axis',(0.,0.,1.));
#127571=DIRECTION('',(1.,0.,0.));
#127572=DIRECTION('center_axis',(-1.,0.,0.));
#127573=DIRECTION('ref_axis',(0.,0.,1.));
#127574=DIRECTION('',(-1.,0.,0.));
#127575=DIRECTION('center_axis',(-1.,0.,0.));
#127576=DIRECTION('ref_axis',(0.,0.,1.));
#127577=DIRECTION('',(1.,0.,0.));
#127578=DIRECTION('center_axis',(-1.,0.,0.));
#127579=DIRECTION('ref_axis',(0.,0.,1.));
#127580=DIRECTION('',(-1.,0.,0.));
#127581=DIRECTION('center_axis',(-1.,0.,0.));
#127582=DIRECTION('ref_axis',(0.,0.,1.));
#127583=DIRECTION('',(-1.,0.,0.));
#127584=DIRECTION('',(1.,0.,0.));
#127585=DIRECTION('center_axis',(-1.,0.,0.));
#127586=DIRECTION('ref_axis',(0.,0.,1.));
#127587=DIRECTION('center_axis',(-1.,0.,0.));
#127588=DIRECTION('ref_axis',(0.,0.,1.));
#127589=DIRECTION('',(1.,0.,0.));
#127590=DIRECTION('center_axis',(-1.,0.,0.));
#127591=DIRECTION('ref_axis',(0.,0.,1.));
#127592=DIRECTION('',(-1.,0.,0.));
#127593=DIRECTION('center_axis',(-1.,0.,0.));
#127594=DIRECTION('ref_axis',(0.,0.,1.));
#127595=DIRECTION('',(1.,0.,0.));
#127596=DIRECTION('center_axis',(-1.,0.,0.));
#127597=DIRECTION('ref_axis',(0.,0.,1.));
#127598=DIRECTION('',(-1.,0.,0.));
#127599=DIRECTION('center_axis',(-1.,0.,0.));
#127600=DIRECTION('ref_axis',(0.,0.,1.));
#127601=DIRECTION('',(-1.,0.,0.));
#127602=DIRECTION('',(1.,0.,0.));
#127603=DIRECTION('center_axis',(-1.,0.,0.));
#127604=DIRECTION('ref_axis',(0.,0.,1.));
#127605=DIRECTION('center_axis',(-1.,0.,0.));
#127606=DIRECTION('ref_axis',(0.,0.,1.));
#127607=DIRECTION('',(1.,0.,0.));
#127608=DIRECTION('center_axis',(-1.,0.,0.));
#127609=DIRECTION('ref_axis',(0.,0.,1.));
#127610=DIRECTION('',(-1.,0.,0.));
#127611=DIRECTION('center_axis',(-1.,0.,0.));
#127612=DIRECTION('ref_axis',(0.,0.,1.));
#127613=DIRECTION('',(-1.,0.,0.));
#127614=DIRECTION('',(1.,0.,0.));
#127615=DIRECTION('center_axis',(-1.,0.,0.));
#127616=DIRECTION('ref_axis',(0.,0.,1.));
#127617=DIRECTION('center_axis',(-1.,0.,0.));
#127618=DIRECTION('ref_axis',(0.,0.,1.));
#127619=DIRECTION('center_axis',(-1.,0.,0.));
#127620=DIRECTION('ref_axis',(0.,0.,1.));
#127621=DIRECTION('center_axis',(-1.,0.,0.));
#127622=DIRECTION('ref_axis',(0.,0.,1.));
#127623=DIRECTION('center_axis',(-1.,0.,0.));
#127624=DIRECTION('ref_axis',(0.,0.,1.));
#127625=DIRECTION('center_axis',(-1.,0.,0.));
#127626=DIRECTION('ref_axis',(0.,0.,1.));
#127627=DIRECTION('center_axis',(-1.,0.,0.));
#127628=DIRECTION('ref_axis',(0.,0.,1.));
#127629=DIRECTION('center_axis',(-1.,0.,0.));
#127630=DIRECTION('ref_axis',(0.,0.,1.));
#127631=DIRECTION('center_axis',(-1.,0.,0.));
#127632=DIRECTION('ref_axis',(0.,0.,1.));
#127633=DIRECTION('center_axis',(-1.,0.,0.));
#127634=DIRECTION('ref_axis',(0.,0.,1.));
#127635=DIRECTION('center_axis',(-1.,0.,0.));
#127636=DIRECTION('ref_axis',(0.,0.,1.));
#127637=DIRECTION('center_axis',(-1.,0.,0.));
#127638=DIRECTION('ref_axis',(0.,0.,1.));
#127639=DIRECTION('center_axis',(-1.,0.,0.));
#127640=DIRECTION('ref_axis',(0.,0.,1.));
#127641=DIRECTION('center_axis',(-1.,0.,0.));
#127642=DIRECTION('ref_axis',(0.,0.,1.));
#127643=DIRECTION('center_axis',(-1.,0.,0.));
#127644=DIRECTION('ref_axis',(0.,0.,1.));
#127645=DIRECTION('center_axis',(-1.,0.,0.));
#127646=DIRECTION('ref_axis',(0.,0.,1.));
#127647=DIRECTION('center_axis',(-1.,0.,0.));
#127648=DIRECTION('ref_axis',(0.,0.,1.));
#127649=DIRECTION('center_axis',(-1.,0.,0.));
#127650=DIRECTION('ref_axis',(0.,0.,1.));
#127651=DIRECTION('center_axis',(-1.,0.,0.));
#127652=DIRECTION('ref_axis',(0.,0.,1.));
#127653=DIRECTION('center_axis',(-1.,0.,0.));
#127654=DIRECTION('ref_axis',(0.,0.,1.));
#127655=DIRECTION('center_axis',(-1.,0.,0.));
#127656=DIRECTION('ref_axis',(0.,0.,1.));
#127657=DIRECTION('center_axis',(-1.,0.,0.));
#127658=DIRECTION('ref_axis',(0.,0.,1.));
#127659=DIRECTION('center_axis',(-1.,0.,0.));
#127660=DIRECTION('ref_axis',(0.,0.,1.));
#127661=DIRECTION('center_axis',(-1.,0.,0.));
#127662=DIRECTION('ref_axis',(0.,0.,1.));
#127663=DIRECTION('center_axis',(-1.,0.,0.));
#127664=DIRECTION('ref_axis',(0.,0.,1.));
#127665=DIRECTION('center_axis',(-1.,0.,0.));
#127666=DIRECTION('ref_axis',(0.,0.,1.));
#127667=DIRECTION('center_axis',(-1.,0.,0.));
#127668=DIRECTION('ref_axis',(0.,0.,1.));
#127669=DIRECTION('center_axis',(-1.,0.,0.));
#127670=DIRECTION('ref_axis',(0.,0.,1.));
#127671=DIRECTION('center_axis',(-1.,0.,0.));
#127672=DIRECTION('ref_axis',(0.,0.,1.));
#127673=DIRECTION('center_axis',(-1.,0.,0.));
#127674=DIRECTION('ref_axis',(0.,0.,1.));
#127675=DIRECTION('center_axis',(-1.,0.,0.));
#127676=DIRECTION('ref_axis',(0.,0.,1.));
#127677=DIRECTION('center_axis',(-1.,0.,0.));
#127678=DIRECTION('ref_axis',(0.,0.,1.));
#127679=DIRECTION('',(1.,0.,0.));
#127680=DIRECTION('center_axis',(-1.,0.,0.));
#127681=DIRECTION('ref_axis',(0.,0.,1.));
#127682=DIRECTION('center_axis',(-1.,0.,0.));
#127683=DIRECTION('ref_axis',(0.,0.,1.));
#127684=DIRECTION('center_axis',(-1.,0.,0.));
#127685=DIRECTION('ref_axis',(0.,0.,1.));
#127686=DIRECTION('center_axis',(1.,0.,0.));
#127687=DIRECTION('ref_axis',(0.,0.,-1.));
#127688=DIRECTION('center_axis',(-1.,0.,0.));
#127689=DIRECTION('ref_axis',(0.,-3.56770963698181E-15,-1.));
#127690=DIRECTION('center_axis',(-1.,0.,0.));
#127691=DIRECTION('ref_axis',(0.,0.,-1.));
#127692=DIRECTION('center_axis',(-1.,0.,0.));
#127693=DIRECTION('ref_axis',(0.,-3.60526447526582E-15,-1.));
#127694=DIRECTION('center_axis',(-1.,0.,0.));
#127695=DIRECTION('ref_axis',(0.,1.20175482508861E-15,-1.));
#127696=DIRECTION('center_axis',(-1.,0.,0.));
#127697=DIRECTION('ref_axis',(0.,-1.20175482508861E-15,-1.));
#127698=DIRECTION('center_axis',(-1.,0.,0.));
#127699=DIRECTION('ref_axis',(0.,0.,-1.));
#127700=DIRECTION('center_axis',(-1.,0.,0.));
#127701=DIRECTION('ref_axis',(0.,0.,-1.));
#127702=DIRECTION('center_axis',(-1.,0.,0.));
#127703=DIRECTION('ref_axis',(0.,-1.20175482508861E-15,-1.));
#127704=DIRECTION('center_axis',(-1.,0.,0.));
#127705=DIRECTION('ref_axis',(0.,0.,-1.));
#127706=DIRECTION('center_axis',(-1.,0.,0.));
#127707=DIRECTION('ref_axis',(0.,0.,1.));
#127708=DIRECTION('',(-1.,0.,0.));
#127709=DIRECTION('center_axis',(-1.,0.,0.));
#127710=DIRECTION('ref_axis',(0.,0.,1.));
#127711=DIRECTION('',(-1.,0.,0.));
#127712=DIRECTION('center_axis',(-1.,0.,0.));
#127713=DIRECTION('ref_axis',(0.,0.,1.));
#127714=DIRECTION('center_axis',(-1.,0.,0.));
#127715=DIRECTION('ref_axis',(0.,0.,1.));
#127716=DIRECTION('',(-1.,0.,0.));
#127717=DIRECTION('center_axis',(-1.,0.,0.));
#127718=DIRECTION('ref_axis',(0.,-0.913545457642603,-0.406736643075796));
#127719=DIRECTION('center_axis',(-1.,0.,0.));
#127720=DIRECTION('ref_axis',(0.,0.,1.));
#127721=DIRECTION('center_axis',(-1.,0.,0.));
#127722=DIRECTION('ref_axis',(0.,0.,1.));
#127723=DIRECTION('center_axis',(-1.,0.,0.));
#127724=DIRECTION('ref_axis',(0.,0.,1.));
#127725=DIRECTION('center_axis',(-1.,0.,0.));
#127726=DIRECTION('ref_axis',(0.,0.,1.));
#127727=DIRECTION('center_axis',(-1.,0.,0.));
#127728=DIRECTION('ref_axis',(0.,0.160274827576825,-0.987072428773704));
#127729=DIRECTION('center_axis',(-1.,0.,0.));
#127730=DIRECTION('ref_axis',(0.,0.,1.));
#127731=DIRECTION('center_axis',(-1.,0.,0.));
#127732=DIRECTION('ref_axis',(0.,0.,1.));
#127733=DIRECTION('center_axis',(-1.,0.,0.));
#127734=DIRECTION('ref_axis',(0.,0.,1.));
#127735=DIRECTION('center_axis',(-1.,0.,0.));
#127736=DIRECTION('ref_axis',(0.,0.,1.));
#127737=DIRECTION('',(-1.,0.,0.));
#127738=DIRECTION('center_axis',(-1.,0.,0.));
#127739=DIRECTION('ref_axis',(0.,0.,1.));
#127740=DIRECTION('',(-1.,0.,0.));
#127741=DIRECTION('center_axis',(-1.,0.,0.));
#127742=DIRECTION('ref_axis',(0.,0.,1.));
#127743=DIRECTION('center_axis',(-1.,0.,0.));
#127744=DIRECTION('ref_axis',(0.,0.,1.));
#127745=DIRECTION('center_axis',(-1.,0.,0.));
#127746=DIRECTION('ref_axis',(0.,0.,1.));
#127747=DIRECTION('center_axis',(-1.,0.,0.));
#127748=DIRECTION('ref_axis',(0.,0.,1.));
#127749=DIRECTION('center_axis',(-1.,0.,0.));
#127750=DIRECTION('ref_axis',(0.,0.0484514595736587,-0.99882553835251));
#127751=DIRECTION('center_axis',(-1.,0.,0.));
#127752=DIRECTION('ref_axis',(0.,0.,1.));
#127753=DIRECTION('',(-1.,0.,0.));
#127754=DIRECTION('center_axis',(-1.,0.,0.));
#127755=DIRECTION('ref_axis',(0.,0.,1.));
#127756=DIRECTION('',(-1.,0.,0.));
#127757=DIRECTION('center_axis',(-1.,0.,0.));
#127758=DIRECTION('ref_axis',(0.,0.499999999999999,-0.866025403784439));
#127759=DIRECTION('center_axis',(-1.,0.,0.));
#127760=DIRECTION('ref_axis',(0.,0.,1.));
#127761=DIRECTION('',(-1.,0.,0.));
#127762=DIRECTION('center_axis',(-1.,0.,0.));
#127763=DIRECTION('ref_axis',(0.,0.,1.));
#127764=DIRECTION('',(-1.,0.,0.));
#127765=DIRECTION('center_axis',(-1.,0.,0.));
#127766=DIRECTION('ref_axis',(0.,0.,1.));
#127767=DIRECTION('center_axis',(-1.,0.,0.));
#127768=DIRECTION('ref_axis',(0.,0.,1.));
#127769=DIRECTION('',(-1.,0.,0.));
#127770=DIRECTION('center_axis',(-1.,0.,0.));
#127771=DIRECTION('ref_axis',(0.,0.809016994374948,-0.587785252292472));
#127772=DIRECTION('center_axis',(-1.,0.,0.));
#127773=DIRECTION('ref_axis',(0.,0.,1.));
#127774=DIRECTION('',(-1.,0.,0.));
#127775=DIRECTION('center_axis',(-1.,0.,0.));
#127776=DIRECTION('ref_axis',(0.,0.,1.));
#127777=DIRECTION('',(-1.,0.,0.));
#127778=DIRECTION('center_axis',(-1.,0.,0.));
#127779=DIRECTION('ref_axis',(0.,-0.669130606358862,-0.743144825477391));
#127780=DIRECTION('center_axis',(-1.,0.,0.));
#127781=DIRECTION('ref_axis',(0.,0.,1.));
#127782=DIRECTION('',(-1.,0.,0.));
#127783=DIRECTION('center_axis',(-1.,0.,0.));
#127784=DIRECTION('ref_axis',(0.,0.,1.));
#127785=DIRECTION('',(-1.,0.,0.));
#127786=DIRECTION('center_axis',(-1.,0.,0.));
#127787=DIRECTION('ref_axis',(0.,-0.309016994374949,-0.951056516295153));
#127788=DIRECTION('center_axis',(-1.,0.,0.));
#127789=DIRECTION('ref_axis',(0.,0.,1.));
#127790=DIRECTION('',(-1.,0.,0.));
#127791=DIRECTION('center_axis',(-1.,0.,0.));
#127792=DIRECTION('ref_axis',(0.,0.,1.));
#127793=DIRECTION('',(-1.,0.,0.));
#127794=DIRECTION('center_axis',(-1.,0.,0.));
#127795=DIRECTION('ref_axis',(0.,0.104528463267655,-0.994521895368273));
#127796=DIRECTION('center_axis',(0.,-1.,0.));
#127797=DIRECTION('ref_axis',(0.,0.,-1.));
#127798=DIRECTION('',(-1.,0.,0.));
#127799=DIRECTION('',(-1.,0.,0.));
#127800=DIRECTION('center_axis',(0.,0.,1.));
#127801=DIRECTION('ref_axis',(1.,0.,0.));
#127802=DIRECTION('center_axis',(0.,0.,-1.));
#127803=DIRECTION('ref_axis',(-1.,0.,0.));
#127804=DIRECTION('center_axis',(1.,0.,0.));
#127805=DIRECTION('ref_axis',(0.,0.,-1.));
#127806=DIRECTION('center_axis',(-1.,0.,0.));
#127807=DIRECTION('ref_axis',(0.,0.,-1.));
#127808=DIRECTION('',(1.,0.,0.));
#127809=DIRECTION('center_axis',(1.,0.,0.));
#127810=DIRECTION('ref_axis',(0.,0.,-1.));
#127811=DIRECTION('center_axis',(1.,0.,0.));
#127812=DIRECTION('ref_axis',(0.,-1.,1.83697019872103E-16));
#127813=DIRECTION('center_axis',(-1.,0.,0.));
#127814=DIRECTION('ref_axis',(0.,8.89160511826737E-16,-1.));
#127815=DIRECTION('',(1.,0.,0.));
#127816=DIRECTION('center_axis',(1.,0.,0.));
#127817=DIRECTION('ref_axis',(0.,0.,-1.));
#127818=DIRECTION('',(1.,0.,0.));
#127819=DIRECTION('center_axis',(0.,0.,-1.));
#127820=DIRECTION('ref_axis',(-1.,0.,0.));
#127821=DIRECTION('',(0.,-1.,0.));
#127822=DIRECTION('',(1.,0.,0.));
#127823=DIRECTION('',(0.,1.,0.));
#127824=DIRECTION('center_axis',(0.,1.,0.));
#127825=DIRECTION('ref_axis',(0.,0.,1.));
#127826=DIRECTION('',(0.,0.,-1.));
#127827=DIRECTION('',(1.,0.,0.));
#127828=DIRECTION('',(0.,0.,1.));
#127829=DIRECTION('center_axis',(0.,0.,1.));
#127830=DIRECTION('ref_axis',(1.,0.,0.));
#127831=DIRECTION('',(0.,1.,0.));
#127832=DIRECTION('',(0.,-1.,0.));
#127833=DIRECTION('center_axis',(1.,0.,0.));
#127834=DIRECTION('ref_axis',(0.,0.,-1.));
#127835=DIRECTION('center_axis',(1.,0.,0.));
#127836=DIRECTION('ref_axis',(0.,0.,-1.));
#271223=CARTESIAN_POINT('',(0.,0.,0.));
#271224=CARTESIAN_POINT('Origin',(-9.8073702912372,3.06591104035337,1.49207703394933));
#271225=CARTESIAN_POINT('',(-9.2313702912372,3.06591104035336,34.4680770339493));
#271226=CARTESIAN_POINT('Origin',(-9.2313702912372,3.06591104035337,1.49207703394933));
#271227=CARTESIAN_POINT('',(-9.8073702912372,3.06591104035336,33.8920770339493));
#271228=CARTESIAN_POINT('Origin',(-9.8073702912372,3.06591104035336,34.4680770339493));
#271229=CARTESIAN_POINT('Origin',(-9.8073702912372,3.06591104035337,1.49207703394933));
#271230=CARTESIAN_POINT('Origin',(-22.7900502912372,3.06591104035337,1.49207703394933));
#271231=CARTESIAN_POINT('',(-22.7900502912372,3.06591104035336,33.8920770339493));
#271232=CARTESIAN_POINT('',(-22.7900502912372,3.06591104035336,33.8920770339493));
#271233=CARTESIAN_POINT('Origin',(-22.7900502912372,3.06591104035337,1.49207703394933));
#271234=CARTESIAN_POINT('Origin',(2.4103097087628,-39.1068178299802,-0.976120122868075));
#271235=CARTESIAN_POINT('',(0.0328697087628034,-42.1293633290516,22.1517542177188));
#271236=CARTESIAN_POINT('',(2.35340786587074,-33.8599370650904,21.750617325498));
#271237=CARTESIAN_POINT('Ctrl Pts',(0.032869708762803,-42.1293633290516,
22.1517542177189));
#271238=CARTESIAN_POINT('Ctrl Pts',(0.0352790378720918,-42.1243919042646,
22.1524039254003));
#271239=CARTESIAN_POINT('Ctrl Pts',(0.0376867650499835,-42.1194196830561,
22.1530521068472));
#271240=CARTESIAN_POINT('Ctrl Pts',(0.986850403300165,-40.1576732102835,
22.4081429612987));
#271241=CARTESIAN_POINT('Ctrl Pts',(1.68188687638377,-38.0910153822988,
22.4207048816548));
#271242=CARTESIAN_POINT('Ctrl Pts',(2.20268963592813,-35.2864204920949,
22.0449936368422));
#271243=CARTESIAN_POINT('Ctrl Pts',(2.2980625106802,-34.5685597403789,21.9142157607324));
#271244=CARTESIAN_POINT('Ctrl Pts',(2.35340786587134,-33.8599370650903,
21.750617325498));
#271245=CARTESIAN_POINT('',(-9.17446844834575,-33.8599370650904,21.750617325498));
#271246=CARTESIAN_POINT('',(2.4103097087628,-33.8599370650904,21.750617325498));
#271247=CARTESIAN_POINT('',(-6.85393029123721,-42.1293633290516,22.1517542177189));
#271248=CARTESIAN_POINT('Ctrl Pts',(-9.17446844834572,-33.8599370650904,
21.750617325498));
#271249=CARTESIAN_POINT('Ctrl Pts',(-9.0531834377728,-35.4128281499478,
22.1091304812741));
#271250=CARTESIAN_POINT('Ctrl Pts',(-8.74406947844718,-36.9665376966092,
22.2993317754169));
#271251=CARTESIAN_POINT('Ctrl Pts',(-7.90182428445088,-39.743167770045,
22.3739423544079));
#271252=CARTESIAN_POINT('Ctrl Pts',(-7.41851411808578,-40.9643975216401,
22.3040017656738));
#271253=CARTESIAN_POINT('Ctrl Pts',(-6.85393029123719,-42.1293633290516,
22.1517542177189));
#271254=CARTESIAN_POINT('',(-3.4105302912372,-42.1293633290516,22.1517542177189));
#271255=CARTESIAN_POINT('Origin',(2.4103097087628,-32.5610768757423,-24.3924448318277));
#271256=CARTESIAN_POINT('',(2.4103097087628,-32.2877498558738,-18.6249498118703));
#271257=CARTESIAN_POINT('',(2.35340786587186,-33.8599370650901,-18.7664632575998));
#271258=CARTESIAN_POINT('Ctrl Pts',(2.41030970876281,-32.2877498558686,
-18.6249498118705));
#271259=CARTESIAN_POINT('Ctrl Pts',(2.41030970876289,-32.7156984306091,
-18.604668925942));
#271260=CARTESIAN_POINT('Ctrl Pts',(2.3994466364292,-33.1452146487367,-18.6320357943675));
#271261=CARTESIAN_POINT('Ctrl Pts',(2.36767303424712,-33.6663772566688,
-18.7243858860329));
#271262=CARTESIAN_POINT('Ctrl Pts',(2.36093683952928,-33.7635387054221,
-18.7442079426758));
#271263=CARTESIAN_POINT('Ctrl Pts',(2.35340786587134,-33.8599370650901,
-18.7664632575998));
#271264=CARTESIAN_POINT('',(-9.17446844834572,-33.8599370650901,-18.7664632575998));
#271265=CARTESIAN_POINT('',(2.4103097087628,-33.8599370650901,-18.7664632575998));
#271266=CARTESIAN_POINT('',(-9.2313702912372,-32.2877498558738,-18.6249498118703));
#271267=CARTESIAN_POINT('Ctrl Pts',(-9.17446844834573,-33.8599370650901,
-18.7664632575998));
#271268=CARTESIAN_POINT('Ctrl Pts',(-9.21458398225969,-33.3463117235494,
-18.6478835040821));
#271269=CARTESIAN_POINT('Ctrl Pts',(-9.23137029123717,-32.8175683814159,
-18.5998412130495));
#271270=CARTESIAN_POINT('Ctrl Pts',(-9.2313702912372,-32.2877498558753,
-18.6249498118702));
#271271=CARTESIAN_POINT('',(-9.2313702912372,-26.9914004601507,-25.9147493646419));
#271272=CARTESIAN_POINT('Origin',(-9.2313702912372,-32.5610768757423,-24.3924448318277));
#271273=CARTESIAN_POINT('',(-9.17446844834575,-27.6118203108419,-27.3662581951399));
#271274=CARTESIAN_POINT('Ctrl Pts',(-9.2313702912372,-26.9914004601507,
-25.9147493646419));
#271275=CARTESIAN_POINT('Ctrl Pts',(-9.2313702912372,-27.0255164279608,
-26.0395699226914));
#271276=CARTESIAN_POINT('Ctrl Pts',(-9.2303894871794,-27.0638636212061,
-26.1633730084678));
#271277=CARTESIAN_POINT('Ctrl Pts',(-9.22181693596821,-27.2377195901812,
-26.6642059035602));
#271278=CARTESIAN_POINT('Ctrl Pts',(-9.20467998252579,-27.4073538643018,
-27.0259688833341));
#271279=CARTESIAN_POINT('Ctrl Pts',(-9.17446844834573,-27.6118203108419,
-27.3662581951399));
#271280=CARTESIAN_POINT('',(2.3534078658721,-27.6118203108419,-27.3662581951399));
#271281=CARTESIAN_POINT('',(2.4103097087628,-27.6118203108419,-27.3662581951399));
#271282=CARTESIAN_POINT('',(2.4103097087628,-26.9914004601507,-25.9147493646419));
#271283=CARTESIAN_POINT('Ctrl Pts',(2.35340786587134,-27.6118203108419,
-27.3662581951399));
#271284=CARTESIAN_POINT('Ctrl Pts',(2.36852800519452,-27.5094898187796,
-27.1959516567818));
#271285=CARTESIAN_POINT('Ctrl Pts',(2.38043097016003,-27.4156364467956,
-27.0198481109634));
#271286=CARTESIAN_POINT('Ctrl Pts',(2.40398237976074,-27.1912363180884,
-26.5400168162761));
#271287=CARTESIAN_POINT('Ctrl Pts',(2.41030970876281,-27.0778295126518,
-26.2309685211646));
#271288=CARTESIAN_POINT('Ctrl Pts',(2.41030970876281,-26.9914004601507,
-25.9147493646419));
#271289=CARTESIAN_POINT('Origin',(2.4103097087628,-32.5610768757423,-24.3924448318277));
#271290=CARTESIAN_POINT('Origin',(2.4103097087628,-18.9527784085753,-36.6454118076767));
#271291=CARTESIAN_POINT('',(2.4103097087628,-13.2454487831566,-35.7707147104817));
#271292=CARTESIAN_POINT('',(2.4103097087628,-21.0489333144974,-31.2653708156951));
#271293=CARTESIAN_POINT('Origin',(2.4103097087628,-18.9527784085753,-36.6454118076767));
#271294=CARTESIAN_POINT('',(2.35340786587055,-22.4276390941746,-32.034115929));
#271295=CARTESIAN_POINT('Ctrl Pts',(2.41030970876281,-21.0489333144974,
-31.2653708156951));
#271296=CARTESIAN_POINT('Ctrl Pts',(2.41030970876281,-21.4481327705155,
-31.4209056711769));
#271297=CARTESIAN_POINT('Ctrl Pts',(2.3994466364291,-21.8293842523733,-31.620606534224));
#271298=CARTESIAN_POINT('Ctrl Pts',(2.36767303424712,-22.2679278192698,
-31.9169484706239));
#271299=CARTESIAN_POINT('Ctrl Pts',(2.36093683952928,-22.3486268626585,
-31.9745759419334));
#271300=CARTESIAN_POINT('Ctrl Pts',(2.35340786587133,-22.4276390941746,
-32.0341159290001));
#271301=CARTESIAN_POINT('',(-9.17446844834572,-22.4276390941746,-32.034115929));
#271302=CARTESIAN_POINT('',(2.4103097087628,-22.4276390941746,-32.034115929));
#271303=CARTESIAN_POINT('',(-9.2313702912372,-21.0489333144974,-31.2653708156951));
#271304=CARTESIAN_POINT('Ctrl Pts',(-9.17446844834573,-22.4276390941746,
-32.034115929));
#271305=CARTESIAN_POINT('Ctrl Pts',(-9.21458398225983,-22.006649727361,
-31.7168776865875));
#271306=CARTESIAN_POINT('Ctrl Pts',(-9.2313702912372,-21.5431592090758,
-31.457929577812));
#271307=CARTESIAN_POINT('Ctrl Pts',(-9.2313702912372,-21.0489333144974,
-31.2653708156951));
#271308=CARTESIAN_POINT('',(-9.2313702912372,-13.2454487831566,-35.7707147104817));
#271309=CARTESIAN_POINT('Origin',(-9.2313702912372,-18.9527784085753,-36.6454118076767));
#271310=CARTESIAN_POINT('',(-9.17446844834574,-13.2218486904752,-37.349081496679));
#271311=CARTESIAN_POINT('Ctrl Pts',(-9.2313702912372,-13.2454487831566,
-35.7707147104817));
#271312=CARTESIAN_POINT('Ctrl Pts',(-9.2313702912372,-13.2258461758147,
-35.8986201785306));
#271313=CARTESIAN_POINT('Ctrl Pts',(-9.2303894871794,-13.2105228285062,
-36.0273171338357));
#271314=CARTESIAN_POINT('Ctrl Pts',(-9.2218169359682,-13.1656410687555,
-36.5555643433858));
#271315=CARTESIAN_POINT('Ctrl Pts',(-9.20467998252573,-13.1734674293567,
-36.9550477455079));
#271316=CARTESIAN_POINT('Ctrl Pts',(-9.17446844834573,-13.2218486904752,
-37.349081496679));
#271317=CARTESIAN_POINT('',(2.3534078658719,-13.2218486904752,-37.349081496679));
#271318=CARTESIAN_POINT('',(2.4103097087628,-13.2218486904752,-37.349081496679));
#271319=CARTESIAN_POINT('Ctrl Pts',(2.35340786587134,-13.2218486904752,
-37.349081496679));
#271320=CARTESIAN_POINT('Ctrl Pts',(2.36852800519451,-13.197635043979,-37.1518771713295));
#271321=CARTESIAN_POINT('Ctrl Pts',(2.38043097016002,-13.1835234873784,
-36.9528249715102));
#271322=CARTESIAN_POINT('Ctrl Pts',(2.40398237976074,-13.1736887391474,
-36.4232055167577));
#271323=CARTESIAN_POINT('Ctrl Pts',(2.41030970876281,-13.195787733277,-36.0947491472211));
#271324=CARTESIAN_POINT('Ctrl Pts',(2.41030970876281,-13.2454487831566,
-35.7707147104817));
#271325=CARTESIAN_POINT('Origin',(2.4103097087628,32.5326690847323,-31.234073221581));
#271326=CARTESIAN_POINT('',(2.4103097087628,33.4644445574145,-25.5357839227184));
#271327=CARTESIAN_POINT('',(2.4103097087628,26.7681985526008,-31.565110907066));
#271328=CARTESIAN_POINT('Origin',(2.4103097087628,32.5326690847323,-31.234073221581));
#271329=CARTESIAN_POINT('',(2.35340786587078,27.0732750858163,-33.1138933272357));
#271330=CARTESIAN_POINT('Ctrl Pts',(2.41030970876281,26.7681985526008,-31.565110907066));
#271331=CARTESIAN_POINT('Ctrl Pts',(2.41030970876281,26.7927615743629,-31.992835064575));
#271332=CARTESIAN_POINT('Ctrl Pts',(2.3994466364291,26.864875194449,-32.417137731216));
#271333=CARTESIAN_POINT('Ctrl Pts',(2.36767303424712,27.0111957091688,-32.9257921426857));
#271334=CARTESIAN_POINT('Ctrl Pts',(2.36093683952928,27.0410653154384,-33.0203493617368));
#271335=CARTESIAN_POINT('Ctrl Pts',(2.35340786587133,27.0732750858163,-33.1138933272358));
#271336=CARTESIAN_POINT('',(-9.17446844834572,27.0732750858163,-33.1138933272357));
#271337=CARTESIAN_POINT('',(2.4103097087628,27.0732750858163,-33.1138933272357));
#271338=CARTESIAN_POINT('',(-9.2313702912372,26.7681985526008,-31.565110907066));
#271339=CARTESIAN_POINT('Ctrl Pts',(-9.17446844834573,27.0732750858163,
-33.1138933272357));
#271340=CARTESIAN_POINT('Ctrl Pts',(-9.21458398225973,26.9016564569488,
-32.6154766384669));
#271341=CARTESIAN_POINT('Ctrl Pts',(-9.2313702912372,26.798608617597,-32.094651594538));
#271342=CARTESIAN_POINT('Ctrl Pts',(-9.2313702912372,26.7681985526008,-31.565110907066));
#271343=CARTESIAN_POINT('',(-9.2313702912372,33.4644445574145,-25.5357839227184));
#271344=CARTESIAN_POINT('Origin',(-9.2313702912372,32.5326690847323,-31.234073221581));
#271345=CARTESIAN_POINT('',(-9.17446844834452,34.9728534042387,-26.0010810610805));
#271346=CARTESIAN_POINT('Ctrl Pts',(-9.2313702912372,33.4644445574145,-25.5357839227184));
#271347=CARTESIAN_POINT('Ctrl Pts',(-9.2313702912372,33.5921474250748,-25.5566656985701));
#271348=CARTESIAN_POINT('Ctrl Pts',(-9.2303894871794,33.7192806777741,-25.5818618755744));
#271349=CARTESIAN_POINT('Ctrl Pts',(-9.22181693596821,34.2355428551313,
-25.7024141504828));
#271350=CARTESIAN_POINT('Ctrl Pts',(-9.20467998252578,34.6130556694415,
-25.8333046219577));
#271351=CARTESIAN_POINT('Ctrl Pts',(-9.17446844834572,34.9728534042388,
-26.0010810610805));
#271352=CARTESIAN_POINT('',(2.35340786587065,34.9728534042387,-26.0010810610805));
#271353=CARTESIAN_POINT('',(2.4103097087628,34.9728534042387,-26.0010810610805));
#271354=CARTESIAN_POINT('Ctrl Pts',(2.35340786587133,34.9728534042387,-26.0010810610805));
#271355=CARTESIAN_POINT('Ctrl Pts',(2.36852800519451,34.7927833738366,-25.9171130268998));
#271356=CARTESIAN_POINT('Ctrl Pts',(2.38043097016002,34.6078341929221,-25.8421816265278));
#271357=CARTESIAN_POINT('Ctrl Pts',(2.40398237976075,34.1071752636619,-25.6691668130665));
#271358=CARTESIAN_POINT('Ctrl Pts',(2.41030970876281,33.7879657283509,-25.5886856053395));
#271359=CARTESIAN_POINT('Ctrl Pts',(2.41030970876281,33.4644445574145,-25.5357839227184));
#271360=CARTESIAN_POINT('Origin',(2.4103097087628,43.296058498978,-16.4195386288221));
#271361=CARTESIAN_POINT('',(2.35340786587189,43.3968281352698,-10.6464500321153));
#271362=CARTESIAN_POINT('',(2.4103097087628,41.8295746888954,-10.8349050956536));
#271363=CARTESIAN_POINT('Ctrl Pts',(2.35340786587134,43.3968281352698,-10.6464500321153));
#271364=CARTESIAN_POINT('Ctrl Pts',(2.36852800519451,43.19817310059,-10.6429824955866));
#271365=CARTESIAN_POINT('Ctrl Pts',(2.38043097016002,42.9987362702226,-10.6497548641268));
#271366=CARTESIAN_POINT('Ctrl Pts',(2.40398237976065,42.4709901151412,-10.6953342993973));
#271367=CARTESIAN_POINT('Ctrl Pts',(2.41030970876272,42.1466430378622,-10.7516452724824));
#271368=CARTESIAN_POINT('Ctrl Pts',(2.41030970876281,41.8295746889017,-10.8349050956519));
#271369=CARTESIAN_POINT('',(2.4103097087628,38.1645977855604,-19.066577996054));
#271370=CARTESIAN_POINT('Origin',(2.4103097087628,43.296058498978,-16.4195386288221));
#271371=CARTESIAN_POINT('',(2.35340786587133,39.0732456291474,-20.3573753358755));
#271372=CARTESIAN_POINT('Ctrl Pts',(2.41030970876281,38.1645977855604,-19.066577996054));
#271373=CARTESIAN_POINT('Ctrl Pts',(2.41030970876281,38.3610083105048,-19.4473327762551));
#271374=CARTESIAN_POINT('Ctrl Pts',(2.3994466364291,38.5994668228463,-19.8056212982767));
#271375=CARTESIAN_POINT('Ctrl Pts',(2.36767303424712,38.9400256522353,-20.2107863104145));
#271376=CARTESIAN_POINT('Ctrl Pts',(2.36093683952928,39.00577278122,-20.2850195649818));
#271377=CARTESIAN_POINT('Ctrl Pts',(2.35340786587133,39.0732456291474,-20.3573753358755));
#271378=CARTESIAN_POINT('',(-9.17446844834689,39.0732456291474,-20.3573753358755));
#271379=CARTESIAN_POINT('',(2.4103097087628,39.0732456291474,-20.3573753358755));
#271380=CARTESIAN_POINT('',(-9.2313702912372,38.1645977855604,-19.066577996054));
#271381=CARTESIAN_POINT('Ctrl Pts',(-9.17446844834573,39.0732456291473,
-20.3573753358754));
#271382=CARTESIAN_POINT('Ctrl Pts',(-9.21458398225972,38.7137398794559,
-19.9718526188323));
#271383=CARTESIAN_POINT('Ctrl Pts',(-9.2313702912372,38.4077623638987,-19.5379685979788));
#271384=CARTESIAN_POINT('Ctrl Pts',(-9.2313702912372,38.1645977855604,-19.066577996054));
#271385=CARTESIAN_POINT('',(-9.2313702912372,41.8295746888954,-10.8349050956536));
#271386=CARTESIAN_POINT('Origin',(-9.2313702912372,43.296058498978,-16.4195386288221));
#271387=CARTESIAN_POINT('',(-9.17446844834574,43.3968281352698,-10.6464500321153));
#271388=CARTESIAN_POINT('Ctrl Pts',(-9.2313702912372,41.829574688899,-10.8349050956526));
#271389=CARTESIAN_POINT('Ctrl Pts',(-9.23137029123718,41.9547304469883,
-10.8020401114265));
#271390=CARTESIAN_POINT('Ctrl Pts',(-9.23038948717938,42.081120660959,-10.7733482120529));
#271391=CARTESIAN_POINT('Ctrl Pts',(-9.22181693596821,42.6017826556463,
-10.6734954502389));
#271392=CARTESIAN_POINT('Ctrl Pts',(-9.20467998252579,42.9998957233396,
-10.6395215510929));
#271393=CARTESIAN_POINT('Ctrl Pts',(-9.17446844834573,43.3968281352698,
-10.6464500321153));
#271394=CARTESIAN_POINT('',(2.4103097087628,43.3968281352698,-10.6464500321153));
#271395=CARTESIAN_POINT('Origin',(2.4103097087628,16.6742095075206,-40.3899591274171));
#271396=CARTESIAN_POINT('',(2.4103097087628,19.8431318188264,-35.5633000499669));
#271397=CARTESIAN_POINT('',(2.4103097087628,11.2734584802515,-38.347755707952));
#271398=CARTESIAN_POINT('Origin',(2.4103097087628,16.6742095075206,-40.3899591274171));
#271399=CARTESIAN_POINT('',(2.35340786587083,10.9222131989692,-39.886724657776));
#271400=CARTESIAN_POINT('Ctrl Pts',(2.41030970876281,11.2734584802515,-38.347755707952));
#271401=CARTESIAN_POINT('Ctrl Pts',(2.41030970876281,11.1219268292206,-38.7484918501837));
#271402=CARTESIAN_POINT('Ctrl Pts',(2.3994466364291,11.0152264570068,-39.165442875713));
#271403=CARTESIAN_POINT('Ctrl Pts',(2.36767303424712,10.9420085107821,-39.6896357177914));
#271404=CARTESIAN_POINT('Ctrl Pts',(2.36093683952928,10.9308358680558,-39.7881670991269));
#271405=CARTESIAN_POINT('Ctrl Pts',(2.35340786587133,10.9222131989692,-39.886724657776));
#271406=CARTESIAN_POINT('',(-9.17446844834572,10.9222131989692,-39.886724657776));
#271407=CARTESIAN_POINT('',(2.4103097087628,10.9222131989692,-39.886724657776));
#271408=CARTESIAN_POINT('',(-9.2313702912372,11.2734584802515,-38.347755707952));
#271409=CARTESIAN_POINT('Ctrl Pts',(-9.17446844834573,10.9222131989692,
-39.886724657776));
#271410=CARTESIAN_POINT('Ctrl Pts',(-9.21458398225962,10.9681561109631,
-39.3615947707445));
#271411=CARTESIAN_POINT('Ctrl Pts',(-9.2313702912372,11.0858558554005,-38.8438840853825));
#271412=CARTESIAN_POINT('Ctrl Pts',(-9.2313702912372,11.2734584802515,-38.347755707952));
#271413=CARTESIAN_POINT('',(-9.2313702912372,19.8431318188264,-35.5633000499669));
#271414=CARTESIAN_POINT('Origin',(-9.2313702912372,16.6742095075206,-40.3899591274171));
#271415=CARTESIAN_POINT('',(-9.17446844834461,21.0318784730203,-36.6018952879149));
#271416=CARTESIAN_POINT('Ctrl Pts',(-9.2313702912372,19.8431318188264,-35.5633000499669));
#271417=CARTESIAN_POINT('Ctrl Pts',(-9.2313702912372,19.951300810094,-35.6343179371471));
#271418=CARTESIAN_POINT('Ctrl Pts',(-9.2303894871794,20.0571946071597,-35.7090455426256));
#271419=CARTESIAN_POINT('Ctrl Pts',(-9.22181693596822,20.479790546625,-36.0291582707414));
#271420=CARTESIAN_POINT('Ctrl Pts',(-9.20467998252584,20.7714277123617,
-36.3022809612165));
#271421=CARTESIAN_POINT('Ctrl Pts',(-9.17446844834572,21.0318784730204,
-36.6018952879149));
#271422=CARTESIAN_POINT('',(2.35340786587133,21.0318784730203,-36.6018952879149));
#271423=CARTESIAN_POINT('',(2.4103097087628,21.0318784730203,-36.6018952879149));
#271424=CARTESIAN_POINT('Ctrl Pts',(2.35340786587133,21.0318784730203,-36.6018952879149));
#271425=CARTESIAN_POINT('Ctrl Pts',(2.36852800519452,20.9015291910372,-36.4519455920175));
#271426=CARTESIAN_POINT('Ctrl Pts',(2.38043097016003,20.7630470531663,-36.3082667425882));
#271427=CARTESIAN_POINT('Ctrl Pts',(2.40398237976075,20.3760438269421,-35.9465735134324));
#271428=CARTESIAN_POINT('Ctrl Pts',(2.41030970876281,20.1171660621841,-35.7432160568577));
#271429=CARTESIAN_POINT('Ctrl Pts',(2.41030970876281,19.8431318188264,-35.5633000499669));
#271430=CARTESIAN_POINT('Origin',(2.4103097087628,-1.5372485021747,-42.3040604945994));
#271431=CARTESIAN_POINT('',(2.4103097087628,3.32088519137438,-39.1836048418737));
#271432=CARTESIAN_POINT('',(2.4103097087628,-5.64044110768385,-38.2417314942451));
#271433=CARTESIAN_POINT('Origin',(2.4103097087628,-1.5372485021747,-42.3040604945994));
#271434=CARTESIAN_POINT('',(2.35340786587068,-6.58727470336698,-39.5047852612049));
#271435=CARTESIAN_POINT('Ctrl Pts',(2.41030970876281,-5.64044110768385,
-38.2417314942451));
#271436=CARTESIAN_POINT('Ctrl Pts',(2.41030970876281,-5.9418662324227,-38.5461887016341));
#271437=CARTESIAN_POINT('Ctrl Pts',(2.3994466364291,-6.20893113323825,-38.8836934658567));
#271438=CARTESIAN_POINT('Ctrl Pts',(2.36767303424712,-6.48902749234103,
-39.3327870340057));
#271439=CARTESIAN_POINT('Ctrl Pts',(2.36093683952928,-6.5393105326355,-39.4182556066633));
#271440=CARTESIAN_POINT('Ctrl Pts',(2.35340786587133,-6.587274703367,-39.504785261205));
#271441=CARTESIAN_POINT('',(-9.17446844834572,-6.58727470336698,-39.5047852612049));
#271442=CARTESIAN_POINT('',(2.4103097087628,-6.58727470336698,-39.5047852612049));
#271443=CARTESIAN_POINT('',(-9.2313702912372,-5.64044110768384,-38.2417314942451));
#271444=CARTESIAN_POINT('Ctrl Pts',(-9.17446844834573,-6.58727470336698,
-39.5047852612049));
#271445=CARTESIAN_POINT('Ctrl Pts',(-9.21458398225973,-6.33171419737343,
-39.0437419040312));
#271446=CARTESIAN_POINT('Ctrl Pts',(-9.2313702912372,-6.01361822422805,
-38.6186624579893));
#271447=CARTESIAN_POINT('Ctrl Pts',(-9.2313702912372,-5.64044110768386,
-38.2417314942451));
#271448=CARTESIAN_POINT('',(-9.2313702912372,3.32088519137438,-39.1836048418737));
#271449=CARTESIAN_POINT('Origin',(-9.2313702912372,-1.5372485021747,-42.3040604945994));
#271450=CARTESIAN_POINT('',(-9.17446844834575,3.98442455700367,-40.6159156274248));
#271451=CARTESIAN_POINT('Ctrl Pts',(-9.2313702912372,3.32088519137438,-39.1836048418737));
#271452=CARTESIAN_POINT('Ctrl Pts',(-9.2313702912372,3.39081690497477,-39.2924792025117));
#271453=CARTESIAN_POINT('Ctrl Pts',(-9.2303894871794,3.45716124687923,-39.4038171545982));
#271454=CARTESIAN_POINT('Ctrl Pts',(-9.22181693596821,3.71302027135661,
-39.8681399370981));
#271455=CARTESIAN_POINT('Ctrl Pts',(-9.20467998252579,3.86835507312333,
-40.2362694521487));
#271456=CARTESIAN_POINT('Ctrl Pts',(-9.17446844834573,3.98442455700367,
-40.6159156274248));
#271457=CARTESIAN_POINT('',(2.35340786587072,3.98442455700367,-40.6159156274248));
#271458=CARTESIAN_POINT('',(2.4103097087628,3.98442455700367,-40.6159156274248));
#271459=CARTESIAN_POINT('Ctrl Pts',(2.35340786587133,3.98442455700368,-40.6159156274248));
#271460=CARTESIAN_POINT('Ctrl Pts',(2.36852800519451,3.92633459848055,-40.4259119344818));
#271461=CARTESIAN_POINT('Ctrl Pts',(2.38043097016002,3.85826432336187,-40.2383290143428));
#271462=CARTESIAN_POINT('Ctrl Pts',(2.40398237976074,3.65183317380175,-39.7504974146935));
#271463=CARTESIAN_POINT('Ctrl Pts',(2.41030970876281,3.49804949695401,-39.4594260609572));
#271464=CARTESIAN_POINT('Ctrl Pts',(2.41030970876281,3.32088519137438,-39.1836048418737));
#271465=CARTESIAN_POINT('Origin',(2.4103097087628,43.803897557122,-9.69038745895935));
#271466=CARTESIAN_POINT('',(2.35340786587183,43.3968281352696,13.6306041000145));
#271467=CARTESIAN_POINT('',(0.0328697087628034,51.5689486443194,12.3036647920732));
#271468=CARTESIAN_POINT('Ctrl Pts',(2.35340786587133,43.3968281352696,13.6306041000145));
#271469=CARTESIAN_POINT('Ctrl Pts',(2.2321228552984,44.9903239005217,13.6584186720598));
#271470=CARTESIAN_POINT('Ctrl Pts',(1.92300889597276,46.5496262384867,13.521429232696));
#271471=CARTESIAN_POINT('Ctrl Pts',(1.08076370197647,49.2810926945741,13.0171155381819));
#271472=CARTESIAN_POINT('Ctrl Pts',(0.597453535611357,50.4610941799812,
12.6947953765867));
#271473=CARTESIAN_POINT('Ctrl Pts',(0.0328697087627933,51.5689486443194,
12.3036647920732));
#271474=CARTESIAN_POINT('',(-6.85393029123721,51.5689486443194,12.3036647920732));
#271475=CARTESIAN_POINT('',(-3.4105302912372,51.5689486443194,12.3036647920732));
#271476=CARTESIAN_POINT('',(-9.17446844834572,43.3968281352696,13.6306041000145));
#271477=CARTESIAN_POINT('Ctrl Pts',(-6.85393029123722,51.5689486443194,
12.3036647920732));
#271478=CARTESIAN_POINT('Ctrl Pts',(-6.8563396203465,51.5642209389144,12.3053339194162));
#271479=CARTESIAN_POINT('Ctrl Pts',(-6.85874734752439,51.5594921371695,
12.3070017194619));
#271480=CARTESIAN_POINT('Ctrl Pts',(-7.80791098577456,49.6936509024402,
12.9643882528227));
#271481=CARTESIAN_POINT('Ctrl Pts',(-8.50294745885817,47.6747662765604,
13.4063579884377));
#271482=CARTESIAN_POINT('Ctrl Pts',(-9.02375021840253,44.8533437535089,
13.6219650014366));
#271483=CARTESIAN_POINT('Ctrl Pts',(-9.1191230931546,44.1239797322133,13.6432965783518));
#271484=CARTESIAN_POINT('Ctrl Pts',(-9.17446844834574,43.3968281352695,
13.6306041000145));
#271485=CARTESIAN_POINT('',(2.4103097087628,43.3968281352696,13.6306041000145));
#271486=CARTESIAN_POINT('Origin',(15.9689897087628,3.06591104035337,1.49207703394933));
#271487=CARTESIAN_POINT('',(2.4103097087628,17.555631534552,5.81207703394933));
#271488=CARTESIAN_POINT('',(2.4103097087628,17.555631534552,-2.82792296605067));
#271489=CARTESIAN_POINT('Origin',(2.4103097087628,3.06591104035337,1.49207703394933));
#271490=CARTESIAN_POINT('',(-22.7900502912372,17.555631534552,-2.82792296605067));
#271491=CARTESIAN_POINT('',(15.9689897087628,17.555631534552,-2.82792296605067));
#271492=CARTESIAN_POINT('',(-22.7900502912372,17.555631534552,5.81207703394933));
#271493=CARTESIAN_POINT('Origin',(-22.7900502912372,3.06591104035337,1.49207703394933));
#271494=CARTESIAN_POINT('',(15.9689897087628,17.555631534552,5.81207703394933));
#271495=CARTESIAN_POINT('Origin',(2.4103097087628,3.06591104035337,1.49207703394933));
#271496=CARTESIAN_POINT('',(2.4103097087628,-5.64044110768439,41.2258855621436));
#271497=CARTESIAN_POINT('',(2.4103097087628,3.32088519137383,42.1677589097724));
#271498=CARTESIAN_POINT('Origin',(2.4103097087628,-1.53724850217529,45.2882145624979));
#271499=CARTESIAN_POINT('',(2.4103097087628,-13.2454487831571,38.7548687783801));
#271500=CARTESIAN_POINT('Origin',(2.4103097087628,3.06591104035337,1.49207703394933));
#271501=CARTESIAN_POINT('',(2.4103097087628,-21.0489333144978,34.2495248835934));
#271502=CARTESIAN_POINT('Origin',(2.4103097087628,-18.9527784085759,39.6295658755751));
#271503=CARTESIAN_POINT('',(2.4103097087628,-26.9914004601511,28.8989034325401));
#271504=CARTESIAN_POINT('Origin',(2.4103097087628,3.06591104035337,1.49207703394933));
#271505=CARTESIAN_POINT('',(2.4103097087628,-32.2877498558741,21.6091038797685));
#271506=CARTESIAN_POINT('Origin',(2.4103097087628,-32.5610768757426,27.3765988997259));
#271507=CARTESIAN_POINT('',(2.4103097087628,-35.5401699166052,14.3040488191824));
#271508=CARTESIAN_POINT('Origin',(2.4103097087628,3.06591104035337,1.49207703394933));
#271509=CARTESIAN_POINT('',(2.4103097087628,-37.4135972503663,5.49026617684987));
#271510=CARTESIAN_POINT('Origin',(2.4103097087628,-40.0091454711921,10.647962939785));
#271511=CARTESIAN_POINT('',(2.4103097087628,-37.4135972503662,-2.50611210895176));
#271512=CARTESIAN_POINT('Origin',(2.4103097087628,3.06591104035337,1.49207703394933));
#271513=CARTESIAN_POINT('',(2.4103097087628,-35.540169916605,-11.3198947512843));
#271514=CARTESIAN_POINT('Origin',(2.4103097087628,-40.009145471192,-7.66380887188698));
#271515=CARTESIAN_POINT('Origin',(2.4103097087628,3.06591104035337,1.49207703394933));
#271516=CARTESIAN_POINT('Origin',(2.4103097087628,3.06591104035337,1.49207703394933));
#271517=CARTESIAN_POINT('Origin',(2.4103097087628,3.06591104035337,1.49207703394933));
#271518=CARTESIAN_POINT('Origin',(2.4103097087628,3.06591104035337,1.49207703394933));
#271519=CARTESIAN_POINT('Origin',(2.4103097087628,3.06591104035337,1.49207703394933));
#271520=CARTESIAN_POINT('Origin',(2.4103097087628,3.06591104035337,1.49207703394933));
#271521=CARTESIAN_POINT('',(2.4103097087628,43.4921152187147,-3.01326686083735));
#271522=CARTESIAN_POINT('Origin',(2.4103097087628,3.06591104035337,1.49207703394933));
#271523=CARTESIAN_POINT('',(2.4103097087628,43.4921152187147,5.997420928736));
#271524=CARTESIAN_POINT('Origin',(2.4103097087628,47.1032899382114,1.49207703394933));
#271525=CARTESIAN_POINT('',(2.4103097087628,41.8295746888953,13.8190591635527));
#271526=CARTESIAN_POINT('Origin',(2.4103097087628,3.06591104035337,1.49207703394933));
#271527=CARTESIAN_POINT('',(2.4103097087628,38.1645977855601,22.0507320639531));
#271528=CARTESIAN_POINT('Origin',(2.4103097087628,43.2960584989777,19.4036926967212));
#271529=CARTESIAN_POINT('',(2.4103097087628,33.4644445574141,28.5199379906174));
#271530=CARTESIAN_POINT('Origin',(2.4103097087628,3.06591104035337,1.49207703394933));
#271531=CARTESIAN_POINT('',(2.4103097087628,26.7681985526003,34.549264974965));
#271532=CARTESIAN_POINT('Origin',(2.4103097087628,32.5326690847319,34.21822728948));
#271533=CARTESIAN_POINT('',(2.4103097087628,19.8431318188259,38.5474541178658));
#271534=CARTESIAN_POINT('Origin',(2.4103097087628,3.06591104035337,1.49207703394933));
#271535=CARTESIAN_POINT('',(2.4103097087628,11.273458480251,41.3319097758507));
#271536=CARTESIAN_POINT('Origin',(2.4103097087628,16.6742095075201,43.374113195316));
#271537=CARTESIAN_POINT('Origin',(2.4103097087628,3.06591104035337,1.49207703394933));
#271538=CARTESIAN_POINT('',(2.4103097087628,20.5619110403534,-2.82792296605067));
#271539=CARTESIAN_POINT('',(2.4103097087628,3.06591104035337,-2.82792296605067));
#271540=CARTESIAN_POINT('',(2.4103097087628,20.5619110403534,5.81207703394933));
#271541=CARTESIAN_POINT('',(2.4103097087628,3.06591104035337,5.81207703394933));
#271542=CARTESIAN_POINT('',(2.4103097087628,20.5619110403534,1.49207703394933));
#271543=CARTESIAN_POINT('Origin',(-22.7900502912372,3.06591104035337,1.49207703394933));
#271544=CARTESIAN_POINT('',(-22.7900502912372,20.5619110403534,-2.82792296605067));
#271545=CARTESIAN_POINT('',(-22.7900502912372,3.06591104035337,-2.82792296605067));
#271546=CARTESIAN_POINT('',(-22.7900502912372,20.5619110403534,5.81207703394933));
#271547=CARTESIAN_POINT('',(-22.7900502912372,20.5619110403534,1.49207703394933));
#271548=CARTESIAN_POINT('',(-22.7900502912372,3.06591104035337,5.81207703394933));
#271549=CARTESIAN_POINT('Origin',(-15.8776902912372,3.06591104035337,1.49207703394933));
#271550=CARTESIAN_POINT('',(0.0328697087628034,-11.8224981078497,48.9027336387577));
#271551=CARTESIAN_POINT('',(2.35340786587133,-6.58727470336753,42.4889393291034));
#271552=CARTESIAN_POINT('Ctrl Pts',(0.0328697087628055,-11.8224981078497,
48.9027336387577));
#271553=CARTESIAN_POINT('Ctrl Pts',(0.035279037872096,-11.8186887484661,
48.8994738894469));
#271554=CARTESIAN_POINT('Ctrl Pts',(0.0376867650499826,-11.8148799903856,
48.8962125270292));
#271555=CARTESIAN_POINT('Ctrl Pts',(0.986850403300172,-10.3126459350247,
47.6090398850055));
#271556=CARTESIAN_POINT('Ctrl Pts',(1.68188687638377,-8.92044660333834,
46.0816193794912));
#271557=CARTESIAN_POINT('Ctrl Pts',(2.20268963592813,-7.32301419132144,
43.7459993062186));
#271558=CARTESIAN_POINT('Ctrl Pts',(2.29806251068019,-6.93985849316234,
43.1250173236278));
#271559=CARTESIAN_POINT('Ctrl Pts',(2.35340786587134,-6.58727470336753,
42.4889393291034));
#271560=CARTESIAN_POINT('',(0.0328697087628034,-12.7563976933524,48.5992912691242));
#271561=CARTESIAN_POINT('Origin',(0.0328697087628034,3.06591104035337,1.49207703394933));
#271562=CARTESIAN_POINT('',(2.35340786587083,-13.2218486904757,40.3332355645775));
#271563=CARTESIAN_POINT('Ctrl Pts',(2.35340786587133,-13.2218486904757,
40.3332355645775));
#271564=CARTESIAN_POINT('Ctrl Pts',(2.2321228552984,-13.4160765549504,41.9150945788249));
#271565=CARTESIAN_POINT('Ctrl Pts',(1.92300889597277,-13.4428290352261,
43.4801741910106));
#271566=CARTESIAN_POINT('Ctrl Pts',(1.08076370197648,-13.2267940150197,
46.2493925235459));
#271567=CARTESIAN_POINT('Ctrl Pts',(0.597453535611382,-13.0295832989177,
47.456621468522));
#271568=CARTESIAN_POINT('Ctrl Pts',(0.0328697087628101,-12.7563976933524,
48.5992912691242));
#271569=CARTESIAN_POINT('Ctrl Pts',(2.41030970876281,-13.2454487831571,
38.7548687783801));
#271570=CARTESIAN_POINT('Ctrl Pts',(2.41030970876281,-13.1805461911692,
39.1783530762096));
#271571=CARTESIAN_POINT('Ctrl Pts',(2.3994466364291,-13.1628664707968,39.6083769762526));
#271572=CARTESIAN_POINT('Ctrl Pts',(2.36767303424712,-13.2002343324775,
40.1363378140511));
#271573=CARTESIAN_POINT('Ctrl Pts',(2.36093683952928,-13.2097916648931,
40.2350389713415));
#271574=CARTESIAN_POINT('Ctrl Pts',(2.35340786587133,-13.2218486904757,
40.3332355645775));
#271575=CARTESIAN_POINT('Ctrl Pts',(2.35340786587133,-6.58727470336753,
42.4889393291034));
#271576=CARTESIAN_POINT('Ctrl Pts',(2.36852800519451,-6.49095016075001,
42.3151652542167));
#271577=CARTESIAN_POINT('Ctrl Pts',(2.38043097016002,-6.38536670236675,
42.1458340769385));
#271578=CARTESIAN_POINT('Ctrl Pts',(2.40398237976074,-6.0820206759904,41.7115822175219));
#271579=CARTESIAN_POINT('Ctrl Pts',(2.41030970876281,-5.87108040414584,
41.458844895496));
#271580=CARTESIAN_POINT('Ctrl Pts',(2.41030970876281,-5.6404411076844,41.2258855621436));
#271581=CARTESIAN_POINT('Origin',(-15.8776902912372,3.06591104035337,1.49207703394933));
#271582=CARTESIAN_POINT('',(2.35340786587079,3.9844245570031,43.6000696953234));
#271583=CARTESIAN_POINT('Ctrl Pts',(2.41030970876281,3.32088519137384,42.1677589097724));
#271584=CARTESIAN_POINT('Ctrl Pts',(2.41030970876281,3.5524232411681,42.5282328040454));
#271585=CARTESIAN_POINT('Ctrl Pts',(2.3994466364291,3.7434809469525,42.9138881944926));
#271586=CARTESIAN_POINT('Ctrl Pts',(2.36767303424712,3.92408472549392,43.4114032982955));
#271587=CARTESIAN_POINT('Ctrl Pts',(2.36093683952928,3.95549904526253,43.5054586095058));
#271588=CARTESIAN_POINT('Ctrl Pts',(2.35340786587133,3.98442455700311,43.6000696953235));
#271589=CARTESIAN_POINT('',(2.35340786587077,10.9222131989687,42.8708787256748));
#271590=CARTESIAN_POINT('Ctrl Pts',(2.35340786587133,10.9222131989687,42.8708787256748));
#271591=CARTESIAN_POINT('Ctrl Pts',(2.36852800519451,10.9395297634634,42.6729494877959));
#271592=CARTESIAN_POINT('Ctrl Pts',(2.38043097016002,10.9671118576574,42.4753130985289));
#271593=CARTESIAN_POINT('Ctrl Pts',(2.40398237976075,11.0676060985989,41.9552223404273));
#271594=CARTESIAN_POINT('Ctrl Pts',(2.41030970876281,11.1575120958356,41.6385381698543));
#271595=CARTESIAN_POINT('Ctrl Pts',(2.41030970876281,11.273458480251,41.3319097758507));
#271596=CARTESIAN_POINT('',(0.0328697087628034,8.74832380494721,50.8595285768044));
#271597=CARTESIAN_POINT('Ctrl Pts',(0.0328697087628022,8.74832380494719,
50.8595285768044));
#271598=CARTESIAN_POINT('Ctrl Pts',(0.0352790378721036,8.75047796841673,
50.8550012415804));
#271599=CARTESIAN_POINT('Ctrl Pts',(0.0376867650500019,8.75263092645877,
50.850472677282));
#271600=CARTESIAN_POINT('Ctrl Pts',(0.986850403300229,9.60144974457407,
49.0635683201677));
#271601=CARTESIAN_POINT('Ctrl Pts',(1.68188687638381,10.2520292311912,47.1019417727825));
#271602=CARTESIAN_POINT('Ctrl Pts',(2.20268963592814,10.7613740869769,44.3185123672612));
#271603=CARTESIAN_POINT('Ctrl Pts',(2.2980625106802,10.8588281075905,43.595373635343));
#271604=CARTESIAN_POINT('Ctrl Pts',(2.35340786587133,10.9222131989687,42.8708787256748));
#271605=CARTESIAN_POINT('',(0.0328697087628034,7.77174294992524,50.9621713607466));
#271606=CARTESIAN_POINT('Origin',(0.0328697087628034,3.06591104035337,1.49207703394933));
#271607=CARTESIAN_POINT('Ctrl Pts',(2.35340786587133,3.98442455700312,43.6000696953235));
#271608=CARTESIAN_POINT('Ctrl Pts',(2.2321228552984,4.45038859893883,45.1241694020084));
#271609=CARTESIAN_POINT('Ctrl Pts',(1.92300889597277,5.06252421970915,46.564821986591));
#271610=CARTESIAN_POINT('Ctrl Pts',(1.08076370197648,6.38622459962975,49.0067594565937));
#271611=CARTESIAN_POINT('Ctrl Pts',(0.597453535611385,7.05740980202667,
50.0294051509654));
#271612=CARTESIAN_POINT('Ctrl Pts',(0.0328697087627989,7.77174294992525,
50.9621713607466));
#271613=CARTESIAN_POINT('Origin',(-15.8776902912372,3.06591104035337,1.49207703394933));
#271614=CARTESIAN_POINT('',(2.35340786587221,21.0318784730198,39.5860493558137));
#271615=CARTESIAN_POINT('Ctrl Pts',(2.41030970876281,19.8431318188259,38.5474541178658));
#271616=CARTESIAN_POINT('Ctrl Pts',(2.41030970876281,20.20127029416,38.78258839746));
#271617=CARTESIAN_POINT('Ctrl Pts',(2.3994466364291,20.5326703723215,39.0571919577339));
#271618=CARTESIAN_POINT('Ctrl Pts',(2.36767303424712,20.9000177570413,39.4382364463109));
#271619=CARTESIAN_POINT('Ctrl Pts',(2.36093683952928,20.966971907716,39.511382893667));
#271620=CARTESIAN_POINT('Ctrl Pts',(2.35340786587134,21.0318784730198,39.5860493558137));
#271621=CARTESIAN_POINT('',(2.35340786587071,27.0732750858158,36.0980473951347));
#271622=CARTESIAN_POINT('Ctrl Pts',(2.35340786587133,27.0732750858159,36.0980473951347));
#271623=CARTESIAN_POINT('Ctrl Pts',(2.36852800519451,27.0085894808706,35.9101867576236));
#271624=CARTESIAN_POINT('Ctrl Pts',(2.38043097016003,26.9534010162137,35.7184182835424));
#271625=CARTESIAN_POINT('Ctrl Pts',(2.40398237976075,26.8336671045001,35.2024170437078));
#271626=CARTESIAN_POINT('Ctrl Pts',(2.41030970876281,26.7869932634364,34.876543594665));
#271627=CARTESIAN_POINT('Ctrl Pts',(2.41030970876281,26.7681985526003,34.549264974965));
#271628=CARTESIAN_POINT('',(0.0328697087628034,28.3366049276465,44.2802426538737));
#271629=CARTESIAN_POINT('Ctrl Pts',(0.0328697087628083,28.3366049276465,
44.2802426538738));
#271630=CARTESIAN_POINT('Ctrl Pts',(0.0352790378720938,28.3367314207681,
44.2752305501264));
#271631=CARTESIAN_POINT('Ctrl Pts',(0.0376867650499842,28.3368563127672,
44.2702178138554));
#271632=CARTESIAN_POINT('Ctrl Pts',(0.986850403300163,28.3854914087078,
42.2925537385122));
#271633=CARTESIAN_POINT('Ctrl Pts',(1.68188687638376,28.1819599466905,40.2359042001166));
#271634=CARTESIAN_POINT('Ctrl Pts',(2.20268963592813,27.515146893427,37.4859456932235));
#271635=CARTESIAN_POINT('Ctrl Pts',(2.29806251068019,27.310048550989,36.7856874682356));
#271636=CARTESIAN_POINT('Ctrl Pts',(2.35340786587133,27.0732750858159,36.0980473951347));
#271637=CARTESIAN_POINT('',(0.0328697087628034,27.4862025048971,44.7712227215677));
#271638=CARTESIAN_POINT('Origin',(0.0328697087628034,3.06591104035337,1.49207703394933));
#271639=CARTESIAN_POINT('Ctrl Pts',(2.35340786587134,21.0318784730198,39.5860493558137));
#271640=CARTESIAN_POINT('Ctrl Pts',(2.23212285529842,22.0774650053648,40.7888590696392));
#271641=CARTESIAN_POINT('Ctrl Pts',(1.9230088959728,23.2226449172723,41.8559827068265));
#271642=CARTESIAN_POINT('Ctrl Pts',(1.08076370197648,25.4251308357786,43.5484061414277));
#271643=CARTESIAN_POINT('Ctrl Pts',(0.597453535611381,26.4542365054499,
44.2096438541936));
#271644=CARTESIAN_POINT('Ctrl Pts',(0.0328697087628023,27.4862025048971,
44.7712227215677));
#271645=CARTESIAN_POINT('Origin',(-15.8776902912372,3.06591104035337,1.49207703394933));
#271646=CARTESIAN_POINT('',(2.35340786587194,34.9728534042383,28.9852351289796));
#271647=CARTESIAN_POINT('Ctrl Pts',(2.41030970876281,33.4644445574141,28.5199379906174));
#271648=CARTESIAN_POINT('Ctrl Pts',(2.41030970876281,33.8872580623168,28.5890758024631));
#271649=CARTESIAN_POINT('Ctrl Pts',(2.3994466364291,34.3016984286661,28.7051460822974));
#271650=CARTESIAN_POINT('Ctrl Pts',(2.36767303424712,34.7922717195002,28.903833901893));
#271651=CARTESIAN_POINT('Ctrl Pts',(2.36093683952928,34.8831887201699,28.9434238001324));
#271652=CARTESIAN_POINT('Ctrl Pts',(2.35340786587134,34.9728534042383,28.9852351289796));
#271653=CARTESIAN_POINT('',(2.35340786587133,39.0732456291471,23.3415294037746));
#271654=CARTESIAN_POINT('Ctrl Pts',(2.35340786587134,39.0732456291471,23.3415294037746));
#271655=CARTESIAN_POINT('Ctrl Pts',(2.36852800519451,38.9377425835071,23.1962201775173));
#271656=CARTESIAN_POINT('Ctrl Pts',(2.38043097016002,38.80932614691,23.0434781299524));
#271657=CARTESIAN_POINT('Ctrl Pts',(2.40398237976074,38.490067163625,22.6207877104763));
#271658=CARTESIAN_POINT('Ctrl Pts',(2.41030970876281,38.3148838153993,22.3420714627706));
#271659=CARTESIAN_POINT('Ctrl Pts',(2.41030970876281,38.1645977855601,22.0507320639531));
#271660=CARTESIAN_POINT('',(0.0328697087628034,43.5553535001861,30.3024941769768));
#271661=CARTESIAN_POINT('Ctrl Pts',(0.0328697087628094,43.5553535001861,
30.3024941769768));
#271662=CARTESIAN_POINT('Ctrl Pts',(0.0352790378720948,43.5534304511498,
30.2978639429776));
#271663=CARTESIAN_POINT('Ctrl Pts',(0.0376867650499853,43.5515056821448,
30.2932337823743));
#271664=CARTESIAN_POINT('Ctrl Pts',(0.986850403300188,42.7915476059866,
28.466766073943));
#271665=CARTESIAN_POINT('Ctrl Pts',(1.68188687638378,41.7690976341429,26.6707069338002));
#271666=CARTESIAN_POINT('Ctrl Pts',(2.20268963592813,40.0414247065458,24.429712133966));
#271667=CARTESIAN_POINT('Ctrl Pts',(2.29806251068019,39.5692373677238,23.873415424655));
#271668=CARTESIAN_POINT('Ctrl Pts',(2.35340786587133,39.0732456291471,23.3415294037746));
#271669=CARTESIAN_POINT('',(0.0328697087628034,42.9781718142661,31.0969166143042));
#271670=CARTESIAN_POINT('Origin',(0.0328697087628034,3.06591104035337,1.49207703394933));
#271671=CARTESIAN_POINT('Ctrl Pts',(2.35340786587134,34.9728534042383,28.9852351289796));
#271672=CARTESIAN_POINT('Ctrl Pts',(2.23212285529841,36.4172710166947,29.658778123242));
#271673=CARTESIAN_POINT('Ctrl Pts',(1.92300889597277,37.8974832093378,30.1678574416503));
#271674=CARTESIAN_POINT('Ctrl Pts',(1.08076370197648,40.5979248421634,30.8181314538232));
#271675=CARTESIAN_POINT('Ctrl Pts',(0.597453535611371,41.8070092596915,
31.0036271772901));
#271676=CARTESIAN_POINT('Ctrl Pts',(0.0328697087628057,42.9781718142661,
31.0969166143042));
#271677=CARTESIAN_POINT('Origin',(-15.8776902912372,3.06591104035337,1.49207703394933));
#271678=CARTESIAN_POINT('',(0.0328697087628034,-42.5287624981535,21.2546889964492));
#271679=CARTESIAN_POINT('Origin',(0.0328697087628034,3.06591104035337,1.49207703394933));
#271680=CARTESIAN_POINT('',(2.35340786587208,-36.6973334821472,15.3777206306443));
#271681=CARTESIAN_POINT('Ctrl Pts',(2.35340786587134,-36.6973334821471,
15.3777206306443));
#271682=CARTESIAN_POINT('Ctrl Pts',(2.23212285529842,-38.0028476319476,
16.291851479574));
#271683=CARTESIAN_POINT('Ctrl Pts',(1.9230088959728,-39.183829350552,17.3192131821901));
#271684=CARTESIAN_POINT('Ctrl Pts',(1.08076370197649,-41.0972039809274,
19.3327272315678));
#271685=CARTESIAN_POINT('Ctrl Pts',(0.597453535611395,-41.8623901985072,
20.2870771907335));
#271686=CARTESIAN_POINT('Ctrl Pts',(0.0328697087628098,-42.5287624981535,
21.2546889964492));
#271687=CARTESIAN_POINT('Ctrl Pts',(2.41030970876281,-35.5401699166052,
14.3040488191824));
#271688=CARTESIAN_POINT('Ctrl Pts',(2.41030970876281,-35.811451770477,14.6356471495685));
#271689=CARTESIAN_POINT('Ctrl Pts',(2.3994466364291,-36.1191917646125,14.9365278952636));
#271690=CARTESIAN_POINT('Ctrl Pts',(2.36767303424712,-36.5365471092219,
15.2620329177462));
#271691=CARTESIAN_POINT('Ctrl Pts',(2.36093683952928,-36.6162914671653,
15.3209744008423));
#271692=CARTESIAN_POINT('Ctrl Pts',(2.35340786587134,-36.6973334821471,
15.3777206306443));
#271693=CARTESIAN_POINT('Ctrl Pts',(2.35340786587133,-33.8599370650904,
21.750617325498));
#271694=CARTESIAN_POINT('Ctrl Pts',(2.36852800519451,-33.6663440609273,
21.7059228588123));
#271695=CARTESIAN_POINT('Ctrl Pts',(2.38043097016003,-33.4698573492114,
21.6710819862382));
#271696=CARTESIAN_POINT('Ctrl Pts',(2.40398237976075,-32.9441672163663,
21.605940806065));
#271697=CARTESIAN_POINT('Ctrl Pts',(2.41030970876281,-32.6152001912929,
21.5935857000344));
#271698=CARTESIAN_POINT('Ctrl Pts',(2.41030970876281,-32.2877498558741,
21.6091038797685));
#271699=CARTESIAN_POINT('Origin',(-15.8776902912372,3.06591104035337,1.49207703394933));
#271700=CARTESIAN_POINT('',(2.35340786587201,-27.6118203108423,30.3504122630382));
#271701=CARTESIAN_POINT('Ctrl Pts',(2.41030970876281,-26.9914004601511,
28.8989034325401));
#271702=CARTESIAN_POINT('Ctrl Pts',(2.41030970876281,-27.1043555737458,
29.3121738515974));
#271703=CARTESIAN_POINT('Ctrl Pts',(2.3994466364291,-27.263110823053,29.7122112222741));
#271704=CARTESIAN_POINT('Ctrl Pts',(2.36767303424712,-27.5119890821949,
30.1793285688391));
#271705=CARTESIAN_POINT('Ctrl Pts',(2.36093683952928,-27.5608655171943,
30.2656092454424));
#271706=CARTESIAN_POINT('Ctrl Pts',(2.35340786587134,-27.6118203108423,
30.3504122630381));
#271707=CARTESIAN_POINT('',(2.35340786587221,-22.427639094175,35.0182699968983));
#271708=CARTESIAN_POINT('Ctrl Pts',(2.35340786587134,-22.427639094175,35.0182699968983));
#271709=CARTESIAN_POINT('Ctrl Pts',(2.36852800519451,-22.2689619619342,
34.8986982012396));
#271710=CARTESIAN_POINT('Ctrl Pts',(2.38043097016002,-22.1036334785118,
34.7869511348269));
#271711=CARTESIAN_POINT('Ctrl Pts',(2.40398237976074,-21.6498869504732,
34.5136242656428));
#271712=CARTESIAN_POINT('Ctrl Pts',(2.41030970876281,-21.354385893355,34.3685343711888));
#271713=CARTESIAN_POINT('Ctrl Pts',(2.41030970876281,-21.0489333144978,
34.2495248835934));
#271714=CARTESIAN_POINT('',(0.0328697087628034,-29.8189788219714,38.748205461446));
#271715=CARTESIAN_POINT('Ctrl Pts',(0.0328697087628022,-29.8189788219714,
38.748205461446));
#271716=CARTESIAN_POINT('Ctrl Pts',(0.0352790378720899,-29.814172939518,
38.746776938318));
#271717=CARTESIAN_POINT('Ctrl Pts',(0.0376867650499825,-29.8093669502727,
38.7453466969716));
#271718=CARTESIAN_POINT('Ctrl Pts',(0.986850403300177,-27.913467573206,
38.1804696134406));
#271719=CARTESIAN_POINT('Ctrl Pts',(1.68188687638377,-26.0203723086328,
37.3513600313804));
#271720=CARTESIAN_POINT('Ctrl Pts',(2.20268963592813,-23.6110629166404,
35.8673992194675));
#271721=CARTESIAN_POINT('Ctrl Pts',(2.2980625106802,-23.0084566420077,35.4559474124384));
#271722=CARTESIAN_POINT('Ctrl Pts',(2.35340786587134,-22.427639094175,35.0182699968983));
#271723=CARTESIAN_POINT('',(0.0328697087628034,-30.54871741541,38.0911458806337));
#271724=CARTESIAN_POINT('Origin',(0.0328697087628034,3.06591104035337,1.49207703394933));
#271725=CARTESIAN_POINT('Ctrl Pts',(2.35340786587134,-27.6118203108423,
30.3504122630381));
#271726=CARTESIAN_POINT('Ctrl Pts',(2.23212285529841,-28.4326563194549,
31.7165127905467));
#271727=CARTESIAN_POINT('Ctrl Pts',(1.92300889597278,-29.0936711538983,
33.1354029470867));
#271728=CARTESIAN_POINT('Ctrl Pts',(1.08076370197647,-30.0226559110164,
35.7530791349006));
#271729=CARTESIAN_POINT('Ctrl Pts',(0.59745353561138,-30.3335192056265,
36.936150478564));
#271730=CARTESIAN_POINT('Ctrl Pts',(0.0328697087628135,-30.5487174154099,
38.0911458806337));
#271731=CARTESIAN_POINT('Origin',(-15.8776902912372,3.06591104035337,1.49207703394933));
#271732=CARTESIAN_POINT('',(0.0328697087628034,-46.6250743114837,1.9830571016429));
#271733=CARTESIAN_POINT('',(2.35340786587075,-38.9074204377757,4.98007899462811));
#271734=CARTESIAN_POINT('Ctrl Pts',(0.0328697087628096,-46.6250743114837,
1.98305710164289));
#271735=CARTESIAN_POINT('Ctrl Pts',(0.0352790378720954,-46.6207969488729,
1.9856726997732));
#271736=CARTESIAN_POINT('Ctrl Pts',(0.0376867650499864,-46.6165182379192,
1.98828722755271));
#271737=CARTESIAN_POINT('Ctrl Pts',(0.98685040330017,-44.9281284564905,
3.01923849382438));
#271738=CARTESIAN_POINT('Ctrl Pts',(1.68188687638377,-43.0452519785497,
3.8712998464458));
#271739=CARTESIAN_POINT('Ctrl Pts',(2.20268963592813,-40.3303115255954,
4.66880205619103));
#271740=CARTESIAN_POINT('Ctrl Pts',(2.29806251068019,-39.6213209423279,
4.84131079385968));
#271741=CARTESIAN_POINT('Ctrl Pts',(2.35340786587133,-38.9074204377758,
4.9800789946281));
#271742=CARTESIAN_POINT('',(0.0328697087628034,-46.6250743114837,1.00109696625507));
#271743=CARTESIAN_POINT('Origin',(0.0328697087628034,3.06591104035337,1.49207703394933));
#271744=CARTESIAN_POINT('',(2.35340786587081,-38.9074204377757,-1.99592492673002));
#271745=CARTESIAN_POINT('Ctrl Pts',(2.35340786587133,-38.9074204377758,
-1.99592492673002));
#271746=CARTESIAN_POINT('Ctrl Pts',(2.23212285529841,-40.4718774720397,
-1.69182528477713));
#271747=CARTESIAN_POINT('Ctrl Pts',(1.92300889597281,-41.9686236067765,
-1.23363220775526));
#271748=CARTESIAN_POINT('Ctrl Pts',(1.08076370197649,-44.5355482543544,
-0.172435168151975));
#271749=CARTESIAN_POINT('Ctrl Pts',(0.597453535611403,-45.6227497463857,
0.388177628579008));
#271750=CARTESIAN_POINT('Ctrl Pts',(0.0328697087628152,-46.6250743114837,
1.00109696625508));
#271751=CARTESIAN_POINT('Ctrl Pts',(2.41030970876281,-37.4135972503662,
-2.50611210895176));
#271752=CARTESIAN_POINT('Ctrl Pts',(2.41030970876281,-37.7962987474624,
-2.31352223103693));
#271753=CARTESIAN_POINT('Ctrl Pts',(2.3994466364291,-38.19981244571,-2.16382312466987));
#271754=CARTESIAN_POINT('Ctrl Pts',(2.36767303424712,-38.7134803451498,
-2.03621320177717));
#271755=CARTESIAN_POINT('Ctrl Pts',(2.36093683952928,-38.810304102094,-2.01480243008215));
#271756=CARTESIAN_POINT('Ctrl Pts',(2.35340786587133,-38.9074204377758,
-1.99592492673001));
#271757=CARTESIAN_POINT('Ctrl Pts',(2.35340786587133,-38.9074204377758,
4.9800789946281));
#271758=CARTESIAN_POINT('Ctrl Pts',(2.36852800519451,-38.7123855508474,
5.01798993624188));
#271759=CARTESIAN_POINT('Ctrl Pts',(2.38043097016002,-38.5187149483196,
5.06607956089376));
#271760=CARTESIAN_POINT('Ctrl Pts',(2.40398237976074,-38.0119778103818,
5.2203875715726));
#271761=CARTESIAN_POINT('Ctrl Pts',(2.41030970876281,-37.70642620456,5.34290356404062));
#271762=CARTESIAN_POINT('Ctrl Pts',(2.41030970876281,-37.4135972503663,
5.49026617684987));
#271763=CARTESIAN_POINT('Origin',(-15.8776902912372,3.06591104035337,1.49207703394933));
#271764=CARTESIAN_POINT('',(0.0328697087628034,-30.5487174154094,-35.1069918127356));
#271765=CARTESIAN_POINT('Ctrl Pts',(0.0328697087628055,-30.5487174154095,
-35.1069918127356));
#271766=CARTESIAN_POINT('Ctrl Pts',(0.0352790378720928,-30.5477990693881,
-35.1020629360817));
#271767=CARTESIAN_POINT('Ctrl Pts',(0.0376867650499851,-30.5468790257237,
-35.0971337736183));
#271768=CARTESIAN_POINT('Ctrl Pts',(0.986850403300176,-30.1832718463553,
-33.1525745982338));
#271769=CARTESIAN_POINT('Ctrl Pts',(1.68188687638377,-29.5565865521619,
-31.1831843571046));
#271770=CARTESIAN_POINT('Ctrl Pts',(2.20268963592813,-28.3325964411273,
-28.631957270833));
#271771=CARTESIAN_POINT('Ctrl Pts',(2.2980625106802,-27.9863881179909,-27.989643711327));
#271772=CARTESIAN_POINT('Ctrl Pts',(2.35340786587134,-27.6118203108419,
-27.3662581951399));
#271773=CARTESIAN_POINT('',(0.0328697087628034,-29.8189788219709,-35.7640513935478));
#271774=CARTESIAN_POINT('Origin',(0.0328697087628034,3.06591104035337,1.49207703394933));
#271775=CARTESIAN_POINT('Ctrl Pts',(2.35340786587133,-22.4276390941746,
-32.0341159290001));
#271776=CARTESIAN_POINT('Ctrl Pts',(2.2321228552984,-23.7004552534809,-32.9932517008816));
#271777=CARTESIAN_POINT('Ctrl Pts',(1.92300889597279,-25.042477716441,-33.7989598345075));
#271778=CARTESIAN_POINT('Ctrl Pts',(1.08076370197648,-27.5487086511453,
-34.9964771851694));
#271779=CARTESIAN_POINT('Ctrl Pts',(0.597453535611387,-28.6928049437295,
-35.4293021676146));
#271780=CARTESIAN_POINT('Ctrl Pts',(0.0328697087628135,-29.8189788219709,
-35.7640513935478));
#271781=CARTESIAN_POINT('Origin',(-15.8776902912372,3.06591104035337,1.49207703394933));
#271782=CARTESIAN_POINT('',(2.35340786587133,-36.697333482147,-12.3935665627462));
#271783=CARTESIAN_POINT('Ctrl Pts',(2.35340786587133,-36.697333482147,-12.3935665627462));
#271784=CARTESIAN_POINT('Ctrl Pts',(2.36852800519451,-36.5345800162395,
-12.2796053590481));
#271785=CARTESIAN_POINT('Ctrl Pts',(2.38043097016002,-36.3772129295191,
-12.156900370153));
#271786=CARTESIAN_POINT('Ctrl Pts',(2.40398237976074,-35.9770482412004,
-11.8098244255128));
#271787=CARTESIAN_POINT('Ctrl Pts',(2.41030970876281,-35.7477447031261,
-11.5736214626667));
#271788=CARTESIAN_POINT('Ctrl Pts',(2.41030970876281,-35.540169916605,-11.3198947512843));
#271789=CARTESIAN_POINT('',(0.0328697087628034,-42.5287624981532,-18.2705349285512));
#271790=CARTESIAN_POINT('Ctrl Pts',(0.0328697087628071,-42.5287624981532,
-18.2705349285512));
#271791=CARTESIAN_POINT('Ctrl Pts',(0.0352790378720939,-42.5259187925725,
-18.2664057006507));
#271792=CARTESIAN_POINT('Ctrl Pts',(0.0376867650499849,-42.5230734198686,
-18.2622769021438));
#271793=CARTESIAN_POINT('Ctrl Pts',(0.986850403300142,-41.3999782615322,
-16.6337260638887));
#271794=CARTESIAN_POINT('Ctrl Pts',(1.68188687638376,-40.0264495820672,
-15.0894944276046));
#271795=CARTESIAN_POINT('Ctrl Pts',(2.20268963592813,-37.870601435138,-13.2566741404465));
#271796=CARTESIAN_POINT('Ctrl Pts',(2.29806251068019,-37.2930719331431,
-12.8107071169351));
#271797=CARTESIAN_POINT('Ctrl Pts',(2.35340786587133,-36.697333482147,-12.3935665627462));
#271798=CARTESIAN_POINT('',(0.0328697087628034,-42.1293633290513,-19.1676001498208));
#271799=CARTESIAN_POINT('Origin',(0.0328697087628034,3.06591104035337,1.49207703394933));
#271800=CARTESIAN_POINT('Ctrl Pts',(2.35340786587134,-33.8599370650901,
-18.7664632575998));
#271801=CARTESIAN_POINT('Ctrl Pts',(2.23212285529841,-35.4128281499475,
-19.1249764133759));
#271802=CARTESIAN_POINT('Ctrl Pts',(1.9230088959728,-36.9665376966088,-19.3151777075188));
#271803=CARTESIAN_POINT('Ctrl Pts',(1.08076370197649,-39.7431677700446,
-19.3897882865098));
#271804=CARTESIAN_POINT('Ctrl Pts',(0.597453535611398,-40.9643975216398,
-19.3198476977757));
#271805=CARTESIAN_POINT('Ctrl Pts',(0.0328697087628097,-42.1293633290513,
-19.1676001498208));
#271806=CARTESIAN_POINT('Origin',(-15.8776902912372,3.06591104035337,1.49207703394933));
#271807=CARTESIAN_POINT('',(0.0328697087628034,-12.7563976933517,-45.6151372012257));
#271808=CARTESIAN_POINT('Ctrl Pts',(0.0328697087628133,-12.7563976933517,
-45.6151372012257));
#271809=CARTESIAN_POINT('Ctrl Pts',(0.0352790378720981,-12.7575634972597,
-45.6102609233694));
#271810=CARTESIAN_POINT('Ctrl Pts',(0.0376867650499855,-12.7587278665428,
-45.6053836939195));
#271811=CARTESIAN_POINT('Ctrl Pts',(0.9868504033002,-13.2174796507227,-43.6810481285951));
#271812=CARTESIAN_POINT('Ctrl Pts',(1.68188687638379,-13.445997322424,-41.6270247466606));
#271813=CARTESIAN_POINT('Ctrl Pts',(2.20268963592814,-13.3655042570831,
-38.7985212016622));
#271814=CARTESIAN_POINT('Ctrl Pts',(2.2980625106802,-13.3104796770793,-38.070922955836));
#271815=CARTESIAN_POINT('Ctrl Pts',(2.35340786587134,-13.2218486904752,
-37.349081496679));
#271816=CARTESIAN_POINT('',(0.0328697087628034,-11.8224981078491,-45.9185795708593));
#271817=CARTESIAN_POINT('Origin',(0.0328697087628034,3.06591104035337,1.49207703394933));
#271818=CARTESIAN_POINT('Ctrl Pts',(2.35340786587133,-6.587274703367,-39.5047852612049));
#271819=CARTESIAN_POINT('Ctrl Pts',(2.2321228552984,-7.35993446000634,-40.8987003607588));
#271820=CARTESIAN_POINT('Ctrl Pts',(1.92300889597277,-8.25822196352803,
-42.180601077935));
#271821=CARTESIAN_POINT('Ctrl Pts',(1.08076370197648,-10.0607036624973,
-44.2939635712348));
#271822=CARTESIAN_POINT('Ctrl Pts',(0.597453535611391,-10.9298418532942,
-45.154714753303));
#271823=CARTESIAN_POINT('Ctrl Pts',(0.032869708762817,-11.8224981078491,
-45.9185795708593));
#271824=CARTESIAN_POINT('Origin',(-15.8776902912372,3.06591104035337,1.49207703394933));
#271825=CARTESIAN_POINT('',(0.0328697087628034,42.9781718142665,-28.112762546405));
#271826=CARTESIAN_POINT('Ctrl Pts',(0.0328697087628044,42.9781718142665,
-28.112762546405));
#271827=CARTESIAN_POINT('Ctrl Pts',(0.0352790378720942,42.9731739452163,
-28.1123644390816));
#271828=CARTESIAN_POINT('Ctrl Pts',(0.0376867650499829,42.9681756144703,
-28.1119646732901));
#271829=CARTESIAN_POINT('Ctrl Pts',(0.986850403300196,40.9962616380186,
-27.9536111544311));
#271830=CARTESIAN_POINT('Ctrl Pts',(1.68188687638377,38.9721534719365,-27.53621624333));
#271831=CARTESIAN_POINT('Ctrl Pts',(2.20268963592813,36.3069604692216,-26.5856071249667));
#271832=CARTESIAN_POINT('Ctrl Pts',(2.29806251068019,35.6319769466131,-26.3084354165599));
#271833=CARTESIAN_POINT('Ctrl Pts',(2.35340786587133,34.9728534042387,-26.0010810610805));
#271834=CARTESIAN_POINT('',(0.0328697087628034,43.5553535001865,-27.3183401090776));
#271835=CARTESIAN_POINT('Origin',(0.0328697087628034,3.06591104035337,1.49207703394933));
#271836=CARTESIAN_POINT('Ctrl Pts',(2.35340786587133,39.0732456291474,-20.3573753358755));
#271837=CARTESIAN_POINT('Ctrl Pts',(2.23212285529841,40.1601726720691,-21.5229618867843));
#271838=CARTESIAN_POINT('Ctrl Pts',(1.92300889597281,41.1017465979602,-22.773413177224));
#271839=CARTESIAN_POINT('Ctrl Pts',(1.0807637019765,42.5546762914754,-25.1407400682357));
#271840=CARTESIAN_POINT('Ctrl Pts',(0.597453535611398,43.1047208406736,
-26.2333263513415));
#271841=CARTESIAN_POINT('Ctrl Pts',(0.0328697087628114,43.5553535001865,
-27.3183401090776));
#271842=CARTESIAN_POINT('Origin',(-15.8776902912372,3.06591104035337,1.49207703394933));
#271843=CARTESIAN_POINT('',(0.0328697087628034,27.4862025048977,-41.7870686536687));
#271844=CARTESIAN_POINT('Ctrl Pts',(0.0328697087628071,27.4862025048977,
-41.7870686536687));
#271845=CARTESIAN_POINT('Ctrl Pts',(0.0352790378720934,27.4817986491653,
-41.7846721480517));
#271846=CARTESIAN_POINT('Ctrl Pts',(0.0376867650499835,27.4773950462125,
-41.7822739395601));
#271847=CARTESIAN_POINT('Ctrl Pts',(0.986850403300234,25.740370168843,-40.8355611304885));
#271848=CARTESIAN_POINT('Ctrl Pts',(1.68188687638379,24.0610251529196,-39.6309729447144));
#271849=CARTESIAN_POINT('Ctrl Pts',(2.20268963592813,22.0128977532289,-37.6785166475666));
#271850=CARTESIAN_POINT('Ctrl Pts',(2.2980625106802,21.5090055123993,-37.1507671602473));
#271851=CARTESIAN_POINT('Ctrl Pts',(2.35340786587133,21.0318784730203,-36.6018952879149));
#271852=CARTESIAN_POINT('',(0.0328697087628034,28.3366049276471,-41.2960885859748));
#271853=CARTESIAN_POINT('Origin',(0.0328697087628034,3.06591104035337,1.49207703394933));
#271854=CARTESIAN_POINT('Ctrl Pts',(2.35340786587133,27.0732750858163,-33.1138933272358));
#271855=CARTESIAN_POINT('Ctrl Pts',(2.2321228552984,27.5921455877354,-34.6208026830141));
#271856=CARTESIAN_POINT('Ctrl Pts',(1.92300889597279,27.9437118105647,-36.1461193972233));
#271857=CARTESIAN_POINT('Ctrl Pts',(1.08076370197649,28.3081505396363,-38.8997398714277));
#271858=CARTESIAN_POINT('Ctrl Pts',(0.597453535611393,28.3662463619963,
-40.1215903809247));
#271859=CARTESIAN_POINT('Ctrl Pts',(0.0328697087628079,28.3366049276471,
-41.2960885859748));
#271860=CARTESIAN_POINT('Origin',(-15.8776902912372,3.06591104035337,1.49207703394933));
#271861=CARTESIAN_POINT('',(0.0328697087628034,51.5689486443196,-9.31951072417391));
#271862=CARTESIAN_POINT('Ctrl Pts',(0.0328697087628049,51.5689486443196,
-9.31951072417391));
#271863=CARTESIAN_POINT('Ctrl Pts',(0.035279037872092,51.5642209389145,
-9.3211798515169));
#271864=CARTESIAN_POINT('Ctrl Pts',(0.0376867650499852,51.5594921371697,
-9.3228476515626));
#271865=CARTESIAN_POINT('Ctrl Pts',(0.98685040330015,49.6936509024404,-9.98023418492342));
#271866=CARTESIAN_POINT('Ctrl Pts',(1.68188687638376,47.6747662765606,-10.4222039205384));
#271867=CARTESIAN_POINT('Ctrl Pts',(2.20268963592813,44.8533437535091,-10.6378109335374));
#271868=CARTESIAN_POINT('Ctrl Pts',(2.2980625106802,44.1239797322136,-10.6591425104526));
#271869=CARTESIAN_POINT('Ctrl Pts',(2.35340786587134,43.3968281352698,-10.6464500321153));
#271870=CARTESIAN_POINT('',(0.0328697087628034,51.7731096363835,-8.35900877372875));
#271871=CARTESIAN_POINT('Origin',(0.0328697087628034,3.06591104035337,1.49207703394933));
#271872=CARTESIAN_POINT('',(2.35340786587192,44.8472209057105,-3.82288853372976));
#271873=CARTESIAN_POINT('Ctrl Pts',(2.35340786587134,44.8472209057105,-3.82288853372974));
#271874=CARTESIAN_POINT('Ctrl Pts',(2.23212285529842,46.3142649294914,-4.44561177609555));
#271875=CARTESIAN_POINT('Ctrl Pts',(1.92300889597281,47.6830398727272,-5.20498325465543));
#271876=CARTESIAN_POINT('Ctrl Pts',(1.08076370197649,49.9732357872253,-6.77668423652894));
#271877=CARTESIAN_POINT('Ctrl Pts',(0.597453535611392,50.9201213637075,
-7.55108819905984));
#271878=CARTESIAN_POINT('Ctrl Pts',(0.0328697087628119,51.7731096363835,
-8.35900877372874));
#271879=CARTESIAN_POINT('Ctrl Pts',(2.41030970876281,43.4921152187147,-3.01326686083735));
#271880=CARTESIAN_POINT('Ctrl Pts',(2.41030970876281,43.8264120827449,-3.28121630318514));
#271881=CARTESIAN_POINT('Ctrl Pts',(2.39944663642909,44.1899838442304,-3.51153934018084));
#271882=CARTESIAN_POINT('Ctrl Pts',(2.36767303424712,44.6658952728075,-3.74315824157946));
#271883=CARTESIAN_POINT('Ctrl Pts',(2.36093683952928,44.7561516486117,-3.78423192756042));
#271884=CARTESIAN_POINT('Ctrl Pts',(2.35340786587134,44.8472209057105,-3.82288853372975));
#271885=CARTESIAN_POINT('Origin',(-15.8776902912372,3.06591104035337,1.49207703394933));
#271886=CARTESIAN_POINT('',(0.0328697087628034,7.77174294992589,-47.9780172928478));
#271887=CARTESIAN_POINT('Ctrl Pts',(0.0328697087628155,7.77174294992591,
-47.9780172928478));
#271888=CARTESIAN_POINT('Ctrl Pts',(0.0352790378721102,7.76869457417527,
-47.97403676653));
#271889=CARTESIAN_POINT('Ctrl Pts',(0.0376867650500066,7.76564712197171,
-47.9700547873736));
#271890=CARTESIAN_POINT('Ctrl Pts',(0.986850403300151,6.56385872535737,
-46.3986779333939));
#271891=CARTESIAN_POINT('Ctrl Pts',(1.68188687638379,5.51965086921625,-44.6151807136072));
#271892=CARTESIAN_POINT('Ctrl Pts',(2.20268963592814,4.44272890660951,-41.9984746689602));
#271893=CARTESIAN_POINT('Ctrl Pts',(2.29806251068019,4.19705549371556,-41.3114000835396));
#271894=CARTESIAN_POINT('Ctrl Pts',(2.35340786587133,3.98442455700369,-40.6159156274248));
#271895=CARTESIAN_POINT('',(0.0328697087628034,8.74832380494785,-47.8753745089056));
#271896=CARTESIAN_POINT('Origin',(0.0328697087628034,3.06591104035337,1.49207703394933));
#271897=CARTESIAN_POINT('Ctrl Pts',(2.35340786587133,10.9222131989692,-39.8867246577761));
#271898=CARTESIAN_POINT('Ctrl Pts',(2.2321228552984,10.7833097363133,-41.4743985009681));
#271899=CARTESIAN_POINT('Ctrl Pts',(1.92300889597278,10.4840792622747,-43.0108395219927));
#271900=CARTESIAN_POINT('Ctrl Pts',(1.08076370197648,9.69701225982446,-45.6746275835432));
#271901=CARTESIAN_POINT('Ctrl Pts',(0.597453535611381,9.25311405987619,
-46.8144732661759));
#271902=CARTESIAN_POINT('Ctrl Pts',(0.0328697087628118,8.74832380494786,
-47.8753745089056));
#271903=CARTESIAN_POINT('Origin',(-16.4313702912372,3.06591104035337,1.49207703394933));
#271904=CARTESIAN_POINT('',(-6.85393029123721,-11.8224981078497,48.9027336387577));
#271905=CARTESIAN_POINT('',(-3.4105302912372,-11.8224981078497,48.9027336387577));
#271906=CARTESIAN_POINT('',(-6.85393029123721,-12.7563976933524,48.5992912691242));
#271907=CARTESIAN_POINT('Origin',(-6.8539302912372,3.06591104035337,1.49207703394933));
#271908=CARTESIAN_POINT('',(-3.4105302912372,-12.7563976933524,48.5992912691242));
#271909=CARTESIAN_POINT('Origin',(-16.4313702912372,3.06591104035337,1.49207703394933));
#271910=CARTESIAN_POINT('',(-6.85393029123721,7.77174294992524,50.9621713607466));
#271911=CARTESIAN_POINT('',(-3.4105302912372,7.77174294992524,50.9621713607466));
#271912=CARTESIAN_POINT('',(-6.85393029123721,8.74832380494721,50.8595285768044));
#271913=CARTESIAN_POINT('',(-3.4105302912372,8.7483238049472,50.8595285768044));
#271914=CARTESIAN_POINT('Origin',(-6.8539302912372,3.06591104035337,1.49207703394933));
#271915=CARTESIAN_POINT('Origin',(-16.4313702912372,3.06591104035337,1.49207703394933));
#271916=CARTESIAN_POINT('',(-6.85393029123721,27.4862025048971,44.7712227215677));
#271917=CARTESIAN_POINT('',(-3.4105302912372,27.4862025048971,44.7712227215677));
#271918=CARTESIAN_POINT('',(-6.8539302912372,28.3366049276465,44.2802426538738));
#271919=CARTESIAN_POINT('',(-3.4105302912372,28.3366049276465,44.2802426538737));
#271920=CARTESIAN_POINT('Origin',(-6.8539302912372,3.06591104035337,1.49207703394933));
#271921=CARTESIAN_POINT('Origin',(-16.4313702912372,3.06591104035337,1.49207703394933));
#271922=CARTESIAN_POINT('',(-6.85393029123721,42.9781718142661,31.0969166143042));
#271923=CARTESIAN_POINT('',(-3.4105302912372,42.9781718142661,31.0969166143043));
#271924=CARTESIAN_POINT('',(-6.8539302912372,43.5553535001861,30.3024941769768));
#271925=CARTESIAN_POINT('',(-3.4105302912372,43.5553535001861,30.3024941769768));
#271926=CARTESIAN_POINT('Origin',(-6.8539302912372,3.06591104035337,1.49207703394933));
#271927=CARTESIAN_POINT('Origin',(-16.4313702912372,3.06591104035337,1.49207703394933));
#271928=CARTESIAN_POINT('',(-6.8539302912372,-42.5287624981535,21.2546889964492));
#271929=CARTESIAN_POINT('Origin',(-6.8539302912372,3.06591104035337,1.49207703394933));
#271930=CARTESIAN_POINT('',(-3.4105302912372,-42.5287624981535,21.2546889964492));
#271931=CARTESIAN_POINT('Origin',(-16.4313702912372,3.06591104035337,1.49207703394933));
#271932=CARTESIAN_POINT('',(-6.8539302912372,-30.5487174154099,38.0911458806337));
#271933=CARTESIAN_POINT('',(-3.4105302912372,-30.54871741541,38.0911458806337));
#271934=CARTESIAN_POINT('',(-6.8539302912372,-29.8189788219714,38.748205461446));
#271935=CARTESIAN_POINT('',(-3.4105302912372,-29.8189788219714,38.748205461446));
#271936=CARTESIAN_POINT('Origin',(-6.8539302912372,3.06591104035337,1.49207703394933));
#271937=CARTESIAN_POINT('Origin',(-16.4313702912372,3.06591104035337,1.49207703394933));
#271938=CARTESIAN_POINT('',(-6.85393029123721,-46.6250743114837,1.98305710164289));
#271939=CARTESIAN_POINT('',(-3.4105302912372,-46.6250743114837,1.98305710164289));
#271940=CARTESIAN_POINT('',(-6.85393029123721,-46.6250743114837,1.00109696625508));
#271941=CARTESIAN_POINT('Origin',(-6.8539302912372,3.06591104035337,1.49207703394933));
#271942=CARTESIAN_POINT('',(-3.4105302912372,-46.6250743114837,1.00109696625508));
#271943=CARTESIAN_POINT('Origin',(-16.4313702912372,3.06591104035337,1.49207703394933));
#271944=CARTESIAN_POINT('',(-6.85393029123721,-30.5487174154095,-35.1069918127355));
#271945=CARTESIAN_POINT('',(-3.4105302912372,-30.5487174154095,-35.1069918127355));
#271946=CARTESIAN_POINT('',(-6.85393029123721,-29.8189788219709,-35.7640513935478));
#271947=CARTESIAN_POINT('Origin',(-6.8539302912372,3.06591104035337,1.49207703394933));
#271948=CARTESIAN_POINT('',(-3.4105302912372,-29.8189788219709,-35.7640513935478));
#271949=CARTESIAN_POINT('Origin',(-16.4313702912372,3.06591104035337,1.49207703394933));
#271950=CARTESIAN_POINT('',(-6.85393029123721,-42.1293633290513,-19.1676001498208));
#271951=CARTESIAN_POINT('',(-3.4105302912372,-42.1293633290513,-19.1676001498208));
#271952=CARTESIAN_POINT('',(-6.85393029123721,-42.5287624981532,-18.2705349285512));
#271953=CARTESIAN_POINT('',(-3.4105302912372,-42.5287624981532,-18.2705349285512));
#271954=CARTESIAN_POINT('Origin',(-6.8539302912372,3.06591104035337,1.49207703394933));
#271955=CARTESIAN_POINT('Origin',(-16.4313702912372,3.06591104035337,1.49207703394933));
#271956=CARTESIAN_POINT('',(-6.85393029123721,-12.7563976933517,-45.6151372012257));
#271957=CARTESIAN_POINT('',(-3.4105302912372,-12.7563976933517,-45.6151372012257));
#271958=CARTESIAN_POINT('',(-6.85393029123721,-11.8224981078491,-45.9185795708593));
#271959=CARTESIAN_POINT('Origin',(-6.8539302912372,3.06591104035337,1.49207703394933));
#271960=CARTESIAN_POINT('',(-3.4105302912372,-11.8224981078491,-45.9185795708593));
#271961=CARTESIAN_POINT('Origin',(-16.4313702912372,3.06591104035337,1.49207703394933));
#271962=CARTESIAN_POINT('',(-6.85393029123721,42.9781718142665,-28.112762546405));
#271963=CARTESIAN_POINT('',(-3.4105302912372,42.9781718142665,-28.112762546405));
#271964=CARTESIAN_POINT('',(-6.85393029123721,43.5553535001865,-27.3183401090776));
#271965=CARTESIAN_POINT('Origin',(-6.8539302912372,3.06591104035337,1.49207703394933));
#271966=CARTESIAN_POINT('',(-3.4105302912372,43.5553535001865,-27.3183401090776));
#271967=CARTESIAN_POINT('Origin',(-16.4313702912372,3.06591104035337,1.49207703394933));
#271968=CARTESIAN_POINT('',(-6.85393029123721,28.3366049276471,-41.2960885859748));
#271969=CARTESIAN_POINT('',(-3.4105302912372,28.3366049276471,-41.2960885859748));
#271970=CARTESIAN_POINT('',(-6.85393029123721,27.4862025048976,-41.7870686536687));
#271971=CARTESIAN_POINT('',(-3.4105302912372,27.4862025048977,-41.7870686536687));
#271972=CARTESIAN_POINT('Origin',(-6.8539302912372,3.06591104035337,1.49207703394933));
#271973=CARTESIAN_POINT('Origin',(-16.4313702912372,3.06591104035337,1.49207703394933));
#271974=CARTESIAN_POINT('',(-6.85393029123721,51.5689486443196,-9.31951072417391));
#271975=CARTESIAN_POINT('',(-3.4105302912372,51.5689486443196,-9.31951072417391));
#271976=CARTESIAN_POINT('',(-6.8539302912372,51.7731096363835,-8.35900877372874));
#271977=CARTESIAN_POINT('Origin',(-6.8539302912372,3.06591104035337,1.49207703394933));
#271978=CARTESIAN_POINT('',(-3.4105302912372,51.7731096363835,-8.35900877372874));
#271979=CARTESIAN_POINT('Origin',(-16.4313702912372,3.06591104035337,1.49207703394933));
#271980=CARTESIAN_POINT('',(-6.85393029123721,8.74832380494785,-47.8753745089056));
#271981=CARTESIAN_POINT('',(-3.4105302912372,8.74832380494785,-47.8753745089056));
#271982=CARTESIAN_POINT('',(-6.85393029123721,7.77174294992591,-47.9780172928478));
#271983=CARTESIAN_POINT('',(-3.4105302912372,7.7717429499259,-47.9780172928478));
#271984=CARTESIAN_POINT('Origin',(-6.8539302912372,3.06591104035337,1.49207703394933));
#271985=CARTESIAN_POINT('Origin',(9.0566297087628,3.06591104035337,1.49207703394933));
#271986=CARTESIAN_POINT('',(-9.17446844834478,-6.58727470336753,42.4889393291034));
#271987=CARTESIAN_POINT('Ctrl Pts',(-9.17446844834572,-6.58727470336757,
42.4889393291035));
#271988=CARTESIAN_POINT('Ctrl Pts',(-9.0531834377728,-7.3599344600069,43.8828544286572));
#271989=CARTESIAN_POINT('Ctrl Pts',(-8.74406947844719,-8.25822196352857,
45.1647551458335));
#271990=CARTESIAN_POINT('Ctrl Pts',(-7.90182428445088,-10.0607036624979,
47.2781176391333));
#271991=CARTESIAN_POINT('Ctrl Pts',(-7.41851411808579,-10.9298418532948,
48.1388688212015));
#271992=CARTESIAN_POINT('Ctrl Pts',(-6.85393029123721,-11.8224981078497,
48.9027336387577));
#271993=CARTESIAN_POINT('',(-9.2313702912372,-5.64044110768439,41.2258855621436));
#271994=CARTESIAN_POINT('Ctrl Pts',(-9.2313702912372,-5.64044110768439,
41.2258855621436));
#271995=CARTESIAN_POINT('Ctrl Pts',(-9.2313702912372,-5.73148089796471,
41.3178411359666));
#271996=CARTESIAN_POINT('Ctrl Pts',(-9.2303894871794,-5.81952391869129,
41.412952322369));
#271997=CARTESIAN_POINT('Ctrl Pts',(-9.22181693596821,-6.16632994440474,
41.8139324556473));
#271998=CARTESIAN_POINT('Ctrl Pts',(-9.20467998252579,-6.39480873797743,
42.1417215362753));
#271999=CARTESIAN_POINT('Ctrl Pts',(-9.17446844834572,-6.58727470336757,
42.4889393291035));
#272000=CARTESIAN_POINT('',(-9.2313702912372,-13.2454487831571,38.7548687783801));
#272001=CARTESIAN_POINT('Origin',(-9.2313702912372,3.06591104035337,1.49207703394933));
#272002=CARTESIAN_POINT('',(-9.17446844834572,-13.2218486904757,40.3332355645775));
#272003=CARTESIAN_POINT('Ctrl Pts',(-9.17446844834573,-13.2218486904757,
40.3332355645775));
#272004=CARTESIAN_POINT('Ctrl Pts',(-9.21458398225973,-13.1576069969014,
39.8100289569889));
#272005=CARTESIAN_POINT('Ctrl Pts',(-9.2313702912372,-13.1650966155822,
39.279160339353));
#272006=CARTESIAN_POINT('Ctrl Pts',(-9.2313702912372,-13.2454487831571,
38.7548687783801));
#272007=CARTESIAN_POINT('Ctrl Pts',(-6.85393029123721,-12.7563976933524,
48.5992912691241));
#272008=CARTESIAN_POINT('Ctrl Pts',(-6.8563396203465,-12.7575634972604,
48.5944149912678));
#272009=CARTESIAN_POINT('Ctrl Pts',(-6.85874734752439,-12.7587278665434,
48.5895377618179));
#272010=CARTESIAN_POINT('Ctrl Pts',(-7.80791098577455,-13.2174796507233,
46.6652021964936));
#272011=CARTESIAN_POINT('Ctrl Pts',(-8.50294745885817,-13.4459973224246,
44.6111788145591));
#272012=CARTESIAN_POINT('Ctrl Pts',(-9.02375021840253,-13.3655042570837,
41.7826752695607));
#272013=CARTESIAN_POINT('Ctrl Pts',(-9.11912309315459,-13.3104796770798,
41.0550770237344));
#272014=CARTESIAN_POINT('Ctrl Pts',(-9.17446844834573,-13.2218486904757,
40.3332355645775));
#272015=CARTESIAN_POINT('Origin',(9.0566297087628,3.06591104035337,1.49207703394933));
#272016=CARTESIAN_POINT('',(-9.17446844834725,3.9844245570031,43.6000696953234));
#272017=CARTESIAN_POINT('',(-9.2313702912372,3.32088519137382,42.1677589097724));
#272018=CARTESIAN_POINT('Ctrl Pts',(-9.17446844834574,3.98442455700307,
43.6000696953233));
#272019=CARTESIAN_POINT('Ctrl Pts',(-9.21458398225973,3.83030496515345,
43.0959672247623));
#272020=CARTESIAN_POINT('Ctrl Pts',(-9.2313702912372,3.6075391385767,42.6140409128762));
#272021=CARTESIAN_POINT('Ctrl Pts',(-9.2313702912372,3.32088519137384,42.1677589097724));
#272022=CARTESIAN_POINT('Ctrl Pts',(-6.85393029123721,7.77174294992524,
50.9621713607466));
#272023=CARTESIAN_POINT('Ctrl Pts',(-6.8563396203465,7.7686945741746,50.9581908344287));
#272024=CARTESIAN_POINT('Ctrl Pts',(-6.8587473475244,7.76564712197105,50.9542088552723));
#272025=CARTESIAN_POINT('Ctrl Pts',(-7.80791098577456,6.5638587253567,49.3828320012926));
#272026=CARTESIAN_POINT('Ctrl Pts',(-8.50294745885817,5.51965086921566,
47.5993347815059));
#272027=CARTESIAN_POINT('Ctrl Pts',(-9.02375021840254,4.44272890660893,
44.9826287368589));
#272028=CARTESIAN_POINT('Ctrl Pts',(-9.1191230931546,4.19705549371495,44.2955541514382));
#272029=CARTESIAN_POINT('Ctrl Pts',(-9.17446844834574,3.98442455700307,
43.6000696953233));
#272030=CARTESIAN_POINT('',(-9.17446844834575,10.9222131989687,42.8708787256748));
#272031=CARTESIAN_POINT('Ctrl Pts',(-9.17446844834573,10.9222131989687,
42.8708787256748));
#272032=CARTESIAN_POINT('Ctrl Pts',(-9.0531834377728,10.7833097363127,44.4585525688669));
#272033=CARTESIAN_POINT('Ctrl Pts',(-8.74406947844717,10.4840792622741,
45.9949935898914));
#272034=CARTESIAN_POINT('Ctrl Pts',(-7.90182428445088,9.69701225982382,
48.658781651442));
#272035=CARTESIAN_POINT('Ctrl Pts',(-7.41851411808578,9.25311405987554,
49.7986273340746));
#272036=CARTESIAN_POINT('Ctrl Pts',(-6.85393029123721,8.74832380494719,
50.8595285768044));
#272037=CARTESIAN_POINT('',(-9.2313702912372,11.273458480251,41.3319097758507));
#272038=CARTESIAN_POINT('Ctrl Pts',(-9.2313702912372,11.273458480251,41.3319097758507));
#272039=CARTESIAN_POINT('Ctrl Pts',(-9.2313702912372,11.2276911947845,41.4529445913066));
#272040=CARTESIAN_POINT('Ctrl Pts',(-9.2303894871794,11.1859450977989,41.5756433063122));
#272041=CARTESIAN_POINT('Ctrl Pts',(-9.22181693596821,11.032215341675,42.0830156043706));
#272042=CARTESIAN_POINT('Ctrl Pts',(-9.20467998252579,10.9568134079305,
42.4753965275548));
#272043=CARTESIAN_POINT('Ctrl Pts',(-9.17446844834573,10.9222131989687,
42.8708787256748));
#272044=CARTESIAN_POINT('Origin',(-9.2313702912372,3.06591104035337,1.49207703394933));
#272045=CARTESIAN_POINT('Origin',(9.0566297087628,3.06591104035337,1.49207703394933));
#272046=CARTESIAN_POINT('',(-9.17446844834697,21.0318784730198,39.5860493558137));
#272047=CARTESIAN_POINT('',(-9.2313702912372,19.8431318188259,38.5474541178658));
#272048=CARTESIAN_POINT('Ctrl Pts',(-9.17446844834573,21.0318784730198,
39.5860493558137));
#272049=CARTESIAN_POINT('Ctrl Pts',(-9.21458398225973,20.6860462733096,
39.1882149190674));
#272050=CARTESIAN_POINT('Ctrl Pts',(-9.2313702912372,20.286522474016,38.8385603504192));
#272051=CARTESIAN_POINT('Ctrl Pts',(-9.2313702912372,19.8431318188259,38.5474541178658));
#272052=CARTESIAN_POINT('Ctrl Pts',(-6.85393029123721,27.4862025048971,
44.7712227215677));
#272053=CARTESIAN_POINT('Ctrl Pts',(-6.8563396203465,27.4817986491647,44.7688262159506));
#272054=CARTESIAN_POINT('Ctrl Pts',(-6.85874734752438,27.477395046212,44.7664280074591));
#272055=CARTESIAN_POINT('Ctrl Pts',(-7.80791098577456,25.7403701688426,
43.8197151983875));
#272056=CARTESIAN_POINT('Ctrl Pts',(-8.50294745885817,24.0610251529191,
42.6151270126134));
#272057=CARTESIAN_POINT('Ctrl Pts',(-9.02375021840253,22.0128977532284,
40.6626707154655));
#272058=CARTESIAN_POINT('Ctrl Pts',(-9.1191230931546,21.5090055123988,40.1349212281462));
#272059=CARTESIAN_POINT('Ctrl Pts',(-9.17446844834573,21.0318784730198,
39.5860493558137));
#272060=CARTESIAN_POINT('',(-9.17446844834461,27.0732750858158,36.0980473951347));
#272061=CARTESIAN_POINT('Ctrl Pts',(-9.17446844834572,27.0732750858159,
36.0980473951348));
#272062=CARTESIAN_POINT('Ctrl Pts',(-9.05318343777279,27.5921455877349,
37.6049567509131));
#272063=CARTESIAN_POINT('Ctrl Pts',(-8.74406947844717,27.9437118105642,
39.1302734651222));
#272064=CARTESIAN_POINT('Ctrl Pts',(-7.90182428445088,28.3081505396358,
41.8838939393267));
#272065=CARTESIAN_POINT('Ctrl Pts',(-7.41851411808578,28.3662463619957,
43.1057444488237));
#272066=CARTESIAN_POINT('Ctrl Pts',(-6.85393029123721,28.3366049276465,
44.2802426538738));
#272067=CARTESIAN_POINT('',(-9.2313702912372,26.7681985526003,34.549264974965));
#272068=CARTESIAN_POINT('Ctrl Pts',(-9.2313702912372,26.7681985526003,34.549264974965));
#272069=CARTESIAN_POINT('Ctrl Pts',(-9.2313702912372,26.7756173513876,34.6784510128945));
#272070=CARTESIAN_POINT('Ctrl Pts',(-9.2303894871794,26.7873864575631,34.8075215339958));
#272071=CARTESIAN_POINT('Ctrl Pts',(-9.22181693596822,26.8533142424535,
35.3335567171668));
#272072=CARTESIAN_POINT('Ctrl Pts',(-9.20467998252585,26.9440268478866,
35.7226832566201));
#272073=CARTESIAN_POINT('Ctrl Pts',(-9.17446844834572,27.0732750858159,
36.0980473951348));
#272074=CARTESIAN_POINT('Origin',(-9.2313702912372,3.06591104035337,1.49207703394933));
#272075=CARTESIAN_POINT('Origin',(9.0566297087628,3.06591104035337,1.49207703394933));
#272076=CARTESIAN_POINT('',(-9.17446844834746,34.9728534042383,28.9852351289796));
#272077=CARTESIAN_POINT('',(-9.2313702912372,33.4644445574141,28.5199379906174));
#272078=CARTESIAN_POINT('Ctrl Pts',(-9.17446844834574,34.9728534042382,
28.9852351289795));
#272079=CARTESIAN_POINT('Ctrl Pts',(-9.21458398225963,34.4951061257856,
28.7624579143744));
#272080=CARTESIAN_POINT('Ctrl Pts',(-9.2313702912372,33.9879056482328,28.6055335403951));
#272081=CARTESIAN_POINT('Ctrl Pts',(-9.2313702912372,33.4644445574141,28.5199379906174));
#272082=CARTESIAN_POINT('Ctrl Pts',(-6.85393029123721,42.9781718142661,
31.0969166143042));
#272083=CARTESIAN_POINT('Ctrl Pts',(-6.8563396203465,42.9731739452159,31.0965185069808));
#272084=CARTESIAN_POINT('Ctrl Pts',(-6.85874734752439,42.9681756144698,
31.0961187411893));
#272085=CARTESIAN_POINT('Ctrl Pts',(-7.80791098577464,40.996261638018,30.9377652223303));
#272086=CARTESIAN_POINT('Ctrl Pts',(-8.5029474588582,38.9721534719359,30.5203703112291));
#272087=CARTESIAN_POINT('Ctrl Pts',(-9.02375021840254,36.3069604692211,
29.5697611928658));
#272088=CARTESIAN_POINT('Ctrl Pts',(-9.1191230931546,35.6319769466126,29.292589484459));
#272089=CARTESIAN_POINT('Ctrl Pts',(-9.17446844834574,34.9728534042382,
28.9852351289795));
#272090=CARTESIAN_POINT('',(-9.17446844834483,39.0732456291471,23.3415294037746));
#272091=CARTESIAN_POINT('Ctrl Pts',(-9.17446844834572,39.0732456291472,
23.3415294037746));
#272092=CARTESIAN_POINT('Ctrl Pts',(-9.0531834377728,40.1601726720688,24.5071159546834));
#272093=CARTESIAN_POINT('Ctrl Pts',(-8.74406947844721,41.1017465979598,
25.7575672451231));
#272094=CARTESIAN_POINT('Ctrl Pts',(-7.90182428445089,42.554676291475,28.1248941361349));
#272095=CARTESIAN_POINT('Ctrl Pts',(-7.4185141180858,43.1047208406732,29.2174804192407));
#272096=CARTESIAN_POINT('Ctrl Pts',(-6.85393029123721,43.5553535001861,
30.3024941769768));
#272097=CARTESIAN_POINT('',(-9.2313702912372,38.1645977855601,22.0507320639531));
#272098=CARTESIAN_POINT('Ctrl Pts',(-9.2313702912372,38.1645977855601,22.0507320639531));
#272099=CARTESIAN_POINT('Ctrl Pts',(-9.2313702912372,38.2239198908931,22.1657318847802));
#272100=CARTESIAN_POINT('Ctrl Pts',(-9.2303894871794,38.2871692148531,22.27885674631));
#272101=CARTESIAN_POINT('Ctrl Pts',(-9.22181693596821,38.5613550278152,
22.7325985525449));
#272102=CARTESIAN_POINT('Ctrl Pts',(-9.20467998252579,38.8024971388486,
23.051187194492));
#272103=CARTESIAN_POINT('Ctrl Pts',(-9.17446844834572,39.0732456291471,
23.3415294037746));
#272104=CARTESIAN_POINT('Origin',(-9.2313702912372,3.06591104035337,1.49207703394933));
#272105=CARTESIAN_POINT('Origin',(9.0566297087628,3.06591104035337,1.49207703394933));
#272106=CARTESIAN_POINT('',(-9.2313702912372,-32.2877498558741,21.6091038797685));
#272107=CARTESIAN_POINT('Ctrl Pts',(-9.2313702912372,-32.2877498558741,
21.6091038797685));
#272108=CARTESIAN_POINT('Ctrl Pts',(-9.2313702912372,-32.4170036748076,
21.6029784195793));
#272109=CARTESIAN_POINT('Ctrl Pts',(-9.2303894871794,-32.5465973406721,
21.6011915101359));
#272110=CARTESIAN_POINT('Ctrl Pts',(-9.22181693596819,-33.0766421781123,
21.611772486401));
#272111=CARTESIAN_POINT('Ctrl Pts',(-9.20467998252573,-33.4731190909123,
21.6613133595047));
#272112=CARTESIAN_POINT('Ctrl Pts',(-9.17446844834573,-33.8599370650904,
21.750617325498));
#272113=CARTESIAN_POINT('',(-9.2313702912372,-35.5401699166052,14.3040488191824));
#272114=CARTESIAN_POINT('Origin',(-9.2313702912372,3.06591104035337,1.49207703394933));
#272115=CARTESIAN_POINT('',(-9.17446844834664,-36.6973334821472,15.3777206306443));
#272116=CARTESIAN_POINT('Ctrl Pts',(-9.17446844834573,-36.6973334821471,
15.3777206306443));
#272117=CARTESIAN_POINT('Ctrl Pts',(-9.21458398225973,-36.2655291156872,
15.0753679582172));
#272118=CARTESIAN_POINT('Ctrl Pts',(-9.2313702912372,-35.876028382572,14.7145816468342));
#272119=CARTESIAN_POINT('Ctrl Pts',(-9.2313702912372,-35.5401699166052,
14.3040488191824));
#272120=CARTESIAN_POINT('Ctrl Pts',(-6.85393029123721,-42.5287624981535,
21.2546889964492));
#272121=CARTESIAN_POINT('Ctrl Pts',(-6.8563396203465,-42.5259187925728,
21.2505597685487));
#272122=CARTESIAN_POINT('Ctrl Pts',(-6.85874734752439,-42.5230734198688,
21.2464309700419));
#272123=CARTESIAN_POINT('Ctrl Pts',(-7.80791098577461,-41.3999782615324,
19.6178801317866));
#272124=CARTESIAN_POINT('Ctrl Pts',(-8.50294745885819,-40.0264495820673,
18.0736484955025));
#272125=CARTESIAN_POINT('Ctrl Pts',(-9.02375021840253,-37.8706014351381,
16.2408282083446));
#272126=CARTESIAN_POINT('Ctrl Pts',(-9.1191230931546,-37.2930719331433,
15.7948611848331));
#272127=CARTESIAN_POINT('Ctrl Pts',(-9.17446844834573,-36.6973334821471,
15.3777206306443));
#272128=CARTESIAN_POINT('Origin',(9.0566297087628,3.06591104035337,1.49207703394933));
#272129=CARTESIAN_POINT('',(-9.17446844834572,-27.6118203108423,30.3504122630382));
#272130=CARTESIAN_POINT('',(-9.2313702912372,-26.9914004601511,28.8989034325401));
#272131=CARTESIAN_POINT('Ctrl Pts',(-9.17446844834573,-27.6118203108423,
30.3504122630382));
#272132=CARTESIAN_POINT('Ctrl Pts',(-9.21458398225983,-27.3403253042799,
29.8985686940558));
#272133=CARTESIAN_POINT('Ctrl Pts',(-9.2313702912372,-27.131243691954,29.4105497774492));
#272134=CARTESIAN_POINT('Ctrl Pts',(-9.2313702912372,-26.9914004601511,
28.8989034325401));
#272135=CARTESIAN_POINT('Ctrl Pts',(-6.85393029123721,-30.5487174154099,
38.0911458806337));
#272136=CARTESIAN_POINT('Ctrl Pts',(-6.85633962034649,-30.5477990693886,
38.0862170039799));
#272137=CARTESIAN_POINT('Ctrl Pts',(-6.85874734752438,-30.5468790257242,
38.0812878415165));
#272138=CARTESIAN_POINT('Ctrl Pts',(-7.80791098577459,-30.1832718463558,
36.136728666132));
#272139=CARTESIAN_POINT('Ctrl Pts',(-8.50294745885818,-29.5565865521623,
34.1673384250027));
#272140=CARTESIAN_POINT('Ctrl Pts',(-9.02375021840253,-28.3325964411277,
31.6161113387312));
#272141=CARTESIAN_POINT('Ctrl Pts',(-9.11912309315459,-27.9863881179913,
30.9737977792253));
#272142=CARTESIAN_POINT('Ctrl Pts',(-9.17446844834573,-27.6118203108423,
30.3504122630382));
#272143=CARTESIAN_POINT('',(-9.17446844834421,-22.427639094175,35.0182699968983));
#272144=CARTESIAN_POINT('Ctrl Pts',(-9.17446844834572,-22.4276390941751,
35.0182699968984));
#272145=CARTESIAN_POINT('Ctrl Pts',(-9.05318343777278,-23.7004552534814,
35.97740576878));
#272146=CARTESIAN_POINT('Ctrl Pts',(-8.74406947844716,-25.0424777164415,
36.7831139024057));
#272147=CARTESIAN_POINT('Ctrl Pts',(-7.90182428445088,-27.5487086511458,
37.9806312530676));
#272148=CARTESIAN_POINT('Ctrl Pts',(-7.41851411808578,-28.69280494373,38.4134562355128));
#272149=CARTESIAN_POINT('Ctrl Pts',(-6.85393029123721,-29.8189788219714,
38.748205461446));
#272150=CARTESIAN_POINT('',(-9.2313702912372,-21.0489333144978,34.2495248835934));
#272151=CARTESIAN_POINT('Ctrl Pts',(-9.2313702912372,-21.0489333144978,
34.2495248835934));
#272152=CARTESIAN_POINT('Ctrl Pts',(-9.2313702912372,-21.1695040027821,
34.2965012616794));
#272153=CARTESIAN_POINT('Ctrl Pts',(-9.2303894871794,-21.2886205091203,
34.3475793312918));
#272154=CARTESIAN_POINT('Ctrl Pts',(-9.2218169359682,-21.7685368919436,
34.5728341919559));
#272155=CARTESIAN_POINT('Ctrl Pts',(-9.20467998252578,-22.1105864862711,
34.7793537201167));
#272156=CARTESIAN_POINT('Ctrl Pts',(-9.17446844834572,-22.4276390941751,
35.0182699968984));
#272157=CARTESIAN_POINT('Origin',(-9.2313702912372,3.06591104035337,1.49207703394933));
#272158=CARTESIAN_POINT('Origin',(9.0566297087628,3.06591104035337,1.49207703394933));
#272159=CARTESIAN_POINT('',(-9.17446844834575,-38.9074204377757,4.98007899462811));
#272160=CARTESIAN_POINT('Ctrl Pts',(-9.17446844834573,-38.9074204377757,
4.98007899462811));
#272161=CARTESIAN_POINT('Ctrl Pts',(-9.0531834377728,-40.4718774720398,
4.67597935267518));
#272162=CARTESIAN_POINT('Ctrl Pts',(-8.74406947844718,-41.9686236067766,
4.21778627565327));
#272163=CARTESIAN_POINT('Ctrl Pts',(-7.90182428445088,-44.5355482543544,
3.15658923604996));
#272164=CARTESIAN_POINT('Ctrl Pts',(-7.41851411808577,-45.6227497463857,
2.59597643931895));
#272165=CARTESIAN_POINT('Ctrl Pts',(-6.85393029123721,-46.6250743114837,
1.98305710164289));
#272166=CARTESIAN_POINT('',(-9.2313702912372,-37.4135972503663,5.49026617684986));
#272167=CARTESIAN_POINT('Ctrl Pts',(-9.2313702912372,-37.4135972503663,
5.49026617684986));
#272168=CARTESIAN_POINT('Ctrl Pts',(-9.2313702912372,-37.5291850404213,
5.43209802610041));
#272169=CARTESIAN_POINT('Ctrl Pts',(-9.2303894871794,-37.6468479436625,
5.37775511047759));
#272170=CARTESIAN_POINT('Ctrl Pts',(-9.22181693596821,-38.1353716680188,
5.17183265542212));
#272171=CARTESIAN_POINT('Ctrl Pts',(-9.20467998252579,-38.5177214391886,
5.05582880644415));
#272172=CARTESIAN_POINT('Ctrl Pts',(-9.17446844834573,-38.9074204377757,
4.98007899462811));
#272173=CARTESIAN_POINT('',(-9.2313702912372,-37.4135972503662,-2.50611210895178));
#272174=CARTESIAN_POINT('Origin',(-9.2313702912372,3.06591104035337,1.49207703394933));
#272175=CARTESIAN_POINT('',(-9.17446844834572,-38.9074204377757,-1.99592492673002));
#272176=CARTESIAN_POINT('Ctrl Pts',(-9.17446844834573,-38.9074204377757,
-1.99592492673002));
#272177=CARTESIAN_POINT('Ctrl Pts',(-9.21458398225963,-38.3899696091993,
-2.09650717875226));
#272178=CARTESIAN_POINT('Ctrl Pts',(-9.2313702912372,-37.8873979705538,
-2.26767765403261));
#272179=CARTESIAN_POINT('Ctrl Pts',(-9.2313702912372,-37.4135972503662,
-2.50611210895176));
#272180=CARTESIAN_POINT('Ctrl Pts',(-6.85393029123721,-46.6250743114837,
1.00109696625508));
#272181=CARTESIAN_POINT('Ctrl Pts',(-6.8563396203465,-46.6207969488729,
0.998481368124769));
#272182=CARTESIAN_POINT('Ctrl Pts',(-6.85874734752438,-46.6165182379192,
0.995866840345263));
#272183=CARTESIAN_POINT('Ctrl Pts',(-7.8079109857745,-44.9281284564905,
-0.0350844259263218));
#272184=CARTESIAN_POINT('Ctrl Pts',(-8.50294745885815,-43.0452519785498,
-0.887145778547745));
#272185=CARTESIAN_POINT('Ctrl Pts',(-9.02375021840252,-40.3303115255954,
-1.68464798829298));
#272186=CARTESIAN_POINT('Ctrl Pts',(-9.11912309315459,-39.6213209423278,
-1.85715672596162));
#272187=CARTESIAN_POINT('Ctrl Pts',(-9.17446844834573,-38.9074204377757,
-1.99592492673003));
#272188=CARTESIAN_POINT('Origin',(9.0566297087628,3.06591104035337,1.49207703394933));
#272189=CARTESIAN_POINT('Ctrl Pts',(-9.17446844834573,-27.6118203108419,
-27.3662581951399));
#272190=CARTESIAN_POINT('Ctrl Pts',(-9.0531834377728,-28.4326563194546,
-28.7323587226485));
#272191=CARTESIAN_POINT('Ctrl Pts',(-8.74406947844717,-29.0936711538979,
-30.1512488791885));
#272192=CARTESIAN_POINT('Ctrl Pts',(-7.90182428445088,-30.022655911016,
-32.7689250670023));
#272193=CARTESIAN_POINT('Ctrl Pts',(-7.41851411808577,-30.3335192056261,
-33.9519964106658));
#272194=CARTESIAN_POINT('Ctrl Pts',(-6.85393029123721,-30.5487174154095,
-35.1069918127356));
#272195=CARTESIAN_POINT('Origin',(-9.2313702912372,3.06591104035337,1.49207703394933));
#272196=CARTESIAN_POINT('Ctrl Pts',(-6.85393029123721,-29.8189788219709,
-35.7640513935478));
#272197=CARTESIAN_POINT('Ctrl Pts',(-6.8563396203465,-29.8141729395174,
-35.7626228704198));
#272198=CARTESIAN_POINT('Ctrl Pts',(-6.85874734752439,-29.8093669502722,
-35.7611926290733));
#272199=CARTESIAN_POINT('Ctrl Pts',(-7.80791098577461,-27.9134675732054,
-35.1963155455424));
#272200=CARTESIAN_POINT('Ctrl Pts',(-8.50294745885819,-26.0203723086323,
-34.3672059634821));
#272201=CARTESIAN_POINT('Ctrl Pts',(-9.02375021840253,-23.6110629166399,
-32.8832451515692));
#272202=CARTESIAN_POINT('Ctrl Pts',(-9.11912309315459,-23.0084566420073,
-32.4717933445401));
#272203=CARTESIAN_POINT('Ctrl Pts',(-9.17446844834573,-22.4276390941746,
-32.034115929));
#272204=CARTESIAN_POINT('Origin',(9.0566297087628,3.06591104035337,1.49207703394933));
#272205=CARTESIAN_POINT('Ctrl Pts',(-6.85393029123721,-42.1293633290513,
-19.1676001498208));
#272206=CARTESIAN_POINT('Ctrl Pts',(-6.8563396203465,-42.1243919042643,
-19.1682498575022));
#272207=CARTESIAN_POINT('Ctrl Pts',(-6.85874734752439,-42.1194196830558,
-19.1688980389491));
#272208=CARTESIAN_POINT('Ctrl Pts',(-7.80791098577457,-40.1576732102832,
-19.4239888934006));
#272209=CARTESIAN_POINT('Ctrl Pts',(-8.50294745885817,-38.0910153822985,
-19.4365508137567));
#272210=CARTESIAN_POINT('Ctrl Pts',(-9.02375021840253,-35.2864204920946,
-19.060839568944));
#272211=CARTESIAN_POINT('Ctrl Pts',(-9.11912309315459,-34.5685597403786,
-18.9300616928343));
#272212=CARTESIAN_POINT('Ctrl Pts',(-9.17446844834573,-33.8599370650901,
-18.7664632575999));
#272213=CARTESIAN_POINT('',(-9.17446844834426,-36.697333482147,-12.3935665627462));
#272214=CARTESIAN_POINT('Ctrl Pts',(-9.17446844834572,-36.6973334821471,
-12.3935665627462));
#272215=CARTESIAN_POINT('Ctrl Pts',(-9.05318343777279,-38.0028476319475,
-13.3076974116759));
#272216=CARTESIAN_POINT('Ctrl Pts',(-8.74406947844718,-39.1838293505519,
-14.3350591142921));
#272217=CARTESIAN_POINT('Ctrl Pts',(-7.90182428445088,-41.0972039809272,
-16.3485731636698));
#272218=CARTESIAN_POINT('Ctrl Pts',(-7.41851411808579,-41.8623901985069,
-17.3029231228355));
#272219=CARTESIAN_POINT('Ctrl Pts',(-6.85393029123721,-42.5287624981532,
-18.2705349285512));
#272220=CARTESIAN_POINT('',(-9.2313702912372,-35.540169916605,-11.3198947512843));
#272221=CARTESIAN_POINT('Ctrl Pts',(-9.2313702912372,-35.540169916605,-11.3198947512843));
#272222=CARTESIAN_POINT('Ctrl Pts',(-9.2313702912372,-35.6221054987989,
-11.4200477908884));
#272223=CARTESIAN_POINT('Ctrl Pts',(-9.2303894871794,-35.7074926545126,
-11.5175503288896));
#272224=CARTESIAN_POINT('Ctrl Pts',(-9.22181693596822,-36.0700250757452,
-11.9043703520391));
#272225=CARTESIAN_POINT('Ctrl Pts',(-9.20467998252585,-36.3721359563108,
-12.1658608037486));
#272226=CARTESIAN_POINT('Ctrl Pts',(-9.17446844834572,-36.6973334821471,
-12.3935665627463));
#272227=CARTESIAN_POINT('Origin',(-9.2313702912372,3.06591104035337,1.49207703394933));
#272228=CARTESIAN_POINT('Origin',(9.0566297087628,3.06591104035337,1.49207703394933));
#272229=CARTESIAN_POINT('Ctrl Pts',(-9.17446844834573,-13.2218486904752,
-37.349081496679));
#272230=CARTESIAN_POINT('Ctrl Pts',(-9.0531834377728,-13.4160765549498,
-38.9309405109264));
#272231=CARTESIAN_POINT('Ctrl Pts',(-8.74406947844719,-13.4428290352255,
-40.4960201231121));
#272232=CARTESIAN_POINT('Ctrl Pts',(-7.90182428445088,-13.2267940150191,
-43.2652384556475));
#272233=CARTESIAN_POINT('Ctrl Pts',(-7.41851411808578,-13.0295832989171,
-44.4724674006236));
#272234=CARTESIAN_POINT('Ctrl Pts',(-6.85393029123721,-12.7563976933517,
-45.6151372012257));
#272235=CARTESIAN_POINT('Origin',(-9.2313702912372,3.06591104035337,1.49207703394933));
#272236=CARTESIAN_POINT('Ctrl Pts',(-6.85393029123721,-11.8224981078491,
-45.9185795708593));
#272237=CARTESIAN_POINT('Ctrl Pts',(-6.8563396203465,-11.8186887484654,
-45.9153198215484));
#272238=CARTESIAN_POINT('Ctrl Pts',(-6.85874734752438,-11.814879990385,
-45.9120584591307));
#272239=CARTESIAN_POINT('Ctrl Pts',(-7.80791098577457,-10.3126459350241,
-44.624885817107));
#272240=CARTESIAN_POINT('Ctrl Pts',(-8.50294745885817,-8.92044660333771,
-43.0974653115927));
#272241=CARTESIAN_POINT('Ctrl Pts',(-9.02375021840253,-7.32301419132085,
-40.76184523832));
#272242=CARTESIAN_POINT('Ctrl Pts',(-9.11912309315459,-6.93985849316177,
-40.1408632557293));
#272243=CARTESIAN_POINT('Ctrl Pts',(-9.17446844834573,-6.58727470336698,
-39.5047852612049));
#272244=CARTESIAN_POINT('Origin',(9.0566297087628,3.06591104035337,1.49207703394933));
#272245=CARTESIAN_POINT('Ctrl Pts',(-9.17446844834572,34.9728534042388,
-26.0010810610805));
#272246=CARTESIAN_POINT('Ctrl Pts',(-9.05318343777278,36.4172710166952,
-26.6746240553429));
#272247=CARTESIAN_POINT('Ctrl Pts',(-8.74406947844716,37.8974832093382,
-27.1837033737512));
#272248=CARTESIAN_POINT('Ctrl Pts',(-7.90182428445088,40.5979248421638,
-27.833977385924));
#272249=CARTESIAN_POINT('Ctrl Pts',(-7.41851411808578,41.8070092596918,
-28.019473109391));
#272250=CARTESIAN_POINT('Ctrl Pts',(-6.85393029123721,42.9781718142665,
-28.112762546405));
#272251=CARTESIAN_POINT('Origin',(-9.2313702912372,3.06591104035337,1.49207703394933));
#272252=CARTESIAN_POINT('Ctrl Pts',(-6.85393029123721,43.5553535001865,
-27.3183401090776));
#272253=CARTESIAN_POINT('Ctrl Pts',(-6.8563396203465,43.5534304511502,-27.3137098750784));
#272254=CARTESIAN_POINT('Ctrl Pts',(-6.85874734752438,43.5515056821452,
-27.3090797144751));
#272255=CARTESIAN_POINT('Ctrl Pts',(-7.80791098577445,42.7915476059871,
-25.482612006044));
#272256=CARTESIAN_POINT('Ctrl Pts',(-8.50294745885813,41.7690976341434,
-23.6865528659012));
#272257=CARTESIAN_POINT('Ctrl Pts',(-9.02375021840253,40.0414247065461,
-21.4455580660668));
#272258=CARTESIAN_POINT('Ctrl Pts',(-9.1191230931546,39.5692373677241,-20.8892613567558));
#272259=CARTESIAN_POINT('Ctrl Pts',(-9.17446844834573,39.0732456291473,
-20.3573753358754));
#272260=CARTESIAN_POINT('Origin',(9.0566297087628,3.06591104035337,1.49207703394933));
#272261=CARTESIAN_POINT('Ctrl Pts',(-6.85393029123721,28.3366049276471,
-41.2960885859748));
#272262=CARTESIAN_POINT('Ctrl Pts',(-6.85633962034649,28.3367314207686,
-41.2910764822274));
#272263=CARTESIAN_POINT('Ctrl Pts',(-6.85874734752437,28.3368563127678,
-41.2860637459564));
#272264=CARTESIAN_POINT('Ctrl Pts',(-7.80791098577455,28.3854914087084,
-39.3083996706132));
#272265=CARTESIAN_POINT('Ctrl Pts',(-8.50294745885815,28.181959946691,-37.2517501322177));
#272266=CARTESIAN_POINT('Ctrl Pts',(-9.02375021840252,27.5151468934274,
-34.5017916253246));
#272267=CARTESIAN_POINT('Ctrl Pts',(-9.11912309315459,27.3100485509895,
-33.8015334003366));
#272268=CARTESIAN_POINT('Ctrl Pts',(-9.17446844834573,27.0732750858163,
-33.1138933272357));
#272269=CARTESIAN_POINT('Ctrl Pts',(-9.17446844834572,21.0318784730204,
-36.6018952879149));
#272270=CARTESIAN_POINT('Ctrl Pts',(-9.05318343777278,22.0774650053655,
-37.8047050017404));
#272271=CARTESIAN_POINT('Ctrl Pts',(-8.74406947844713,23.222644917273,-38.8718286389277));
#272272=CARTESIAN_POINT('Ctrl Pts',(-7.90182428445086,25.4251308357792,
-40.5642520735287));
#272273=CARTESIAN_POINT('Ctrl Pts',(-7.41851411808576,26.4542365054505,
-41.2254897862947));
#272274=CARTESIAN_POINT('Ctrl Pts',(-6.85393029123721,27.4862025048976,
-41.7870686536687));
#272275=CARTESIAN_POINT('Origin',(-9.2313702912372,3.06591104035337,1.49207703394933));
#272276=CARTESIAN_POINT('Origin',(9.0566297087628,3.06591104035337,1.49207703394933));
#272277=CARTESIAN_POINT('Ctrl Pts',(-9.17446844834573,43.3968281352698,
-10.6464500321153));
#272278=CARTESIAN_POINT('Ctrl Pts',(-9.0531834377728,44.9903239005218,-10.6742646041606));
#272279=CARTESIAN_POINT('Ctrl Pts',(-8.7440694784472,46.5496262384867,-10.5372751647968));
#272280=CARTESIAN_POINT('Ctrl Pts',(-7.90182428445089,49.2810926945742,
-10.0329614702827));
#272281=CARTESIAN_POINT('Ctrl Pts',(-7.41851411808579,50.4610941799812,
-9.71064130868742));
#272282=CARTESIAN_POINT('Ctrl Pts',(-6.8539302912372,51.5689486443196,-9.31951072417391));
#272283=CARTESIAN_POINT('',(-9.2313702912372,43.4921152187147,-3.01326686083733));
#272284=CARTESIAN_POINT('Origin',(-9.2313702912372,3.06591104035337,1.49207703394933));
#272285=CARTESIAN_POINT('',(-9.17446844834572,44.8472209057105,-3.82288853372976));
#272286=CARTESIAN_POINT('Ctrl Pts',(-9.17446844834573,44.8472209057105,
-3.82288853372977));
#272287=CARTESIAN_POINT('Ctrl Pts',(-9.21458398225962,44.3619898453251,
-3.61692016855346));
#272288=CARTESIAN_POINT('Ctrl Pts',(-9.2313702912372,43.9059889457207,-3.34499965969369));
#272289=CARTESIAN_POINT('Ctrl Pts',(-9.2313702912372,43.4921152187147,-3.01326686083734));
#272290=CARTESIAN_POINT('Ctrl Pts',(-6.85393029123721,51.7731096363835,
-8.35900877372875));
#272291=CARTESIAN_POINT('Ctrl Pts',(-6.8563396203465,51.769469557838,-8.35556101900044));
#272292=CARTESIAN_POINT('Ctrl Pts',(-6.85874734752439,51.7658279378758,
-8.35211403089695));
#272293=CARTESIAN_POINT('Ctrl Pts',(-7.80791098577456,50.328680344989,-6.99265554910357));
#272294=CARTESIAN_POINT('Ctrl Pts',(-8.50294745885818,48.6641027521171,
-5.76774174922925));
#272295=CARTESIAN_POINT('Ctrl Pts',(-9.02375021840253,46.1743002947837,
-4.4231990161438));
#272296=CARTESIAN_POINT('Ctrl Pts',(-9.11912309315459,45.5166694401473,
-4.1070525773466));
#272297=CARTESIAN_POINT('Ctrl Pts',(-9.17446844834573,44.8472209057105,
-3.82288853372976));
#272298=CARTESIAN_POINT('Origin',(9.0566297087628,3.06591104035337,1.49207703394933));
#272299=CARTESIAN_POINT('Ctrl Pts',(-6.85393029123721,8.74832380494786,
-47.8753745089056));
#272300=CARTESIAN_POINT('Ctrl Pts',(-6.8563396203465,8.75047796841738,-47.8708471736816));
#272301=CARTESIAN_POINT('Ctrl Pts',(-6.85874734752438,8.75263092645941,
-47.8663186093833));
#272302=CARTESIAN_POINT('Ctrl Pts',(-7.80791098577455,9.60144974457463,
-46.0794142522692));
#272303=CARTESIAN_POINT('Ctrl Pts',(-8.50294745885816,10.2520292311917,
-44.1177877048839));
#272304=CARTESIAN_POINT('Ctrl Pts',(-9.02375021840252,10.7613740869774,
-41.3343582993625));
#272305=CARTESIAN_POINT('Ctrl Pts',(-9.11912309315459,10.858828107591,-40.6112195674443));
#272306=CARTESIAN_POINT('Ctrl Pts',(-9.17446844834573,10.9222131989692,
-39.886724657776));
#272307=CARTESIAN_POINT('Ctrl Pts',(-9.17446844834573,3.98442455700367,
-40.6159156274248));
#272308=CARTESIAN_POINT('Ctrl Pts',(-9.0531834377728,4.4503885989394,-42.1400153341097));
#272309=CARTESIAN_POINT('Ctrl Pts',(-8.7440694784472,5.06252421970969,-43.5806679186922));
#272310=CARTESIAN_POINT('Ctrl Pts',(-7.90182428445087,6.3862245996304,-46.022605388695));
#272311=CARTESIAN_POINT('Ctrl Pts',(-7.41851411808577,7.05740980202734,
-47.0452510830667));
#272312=CARTESIAN_POINT('Ctrl Pts',(-6.85393029123721,7.77174294992592,
-47.9780172928478));
#272313=CARTESIAN_POINT('Origin',(-9.2313702912372,3.06591104035337,1.49207703394933));
#272314=CARTESIAN_POINT('Origin',(-15.8776902912372,3.06591104035337,1.49207703394933));
#272315=CARTESIAN_POINT('Ctrl Pts',(2.41030970876281,41.8295746888953,13.8190591635527));
#272316=CARTESIAN_POINT('Ctrl Pts',(2.41030970876281,42.2439549272288,13.7102459518845));
#272317=CARTESIAN_POINT('Ctrl Pts',(2.39944663642909,42.6697750773516,13.6477133454304));
#272318=CARTESIAN_POINT('Ctrl Pts',(2.36767303424711,43.1987496955963,13.6296895670144));
#272319=CARTESIAN_POINT('Ctrl Pts',(2.36093683952928,43.2979091708901,13.6288774630686));
#272320=CARTESIAN_POINT('Ctrl Pts',(2.35340786587134,43.3968281352696,13.6306041000145));
#272321=CARTESIAN_POINT('',(2.35340786587067,44.8472209057105,6.80704260162841));
#272322=CARTESIAN_POINT('Ctrl Pts',(2.35340786587133,44.8472209057106,6.80704260162844));
#272323=CARTESIAN_POINT('Ctrl Pts',(2.36852800519451,44.6643301269736,6.72941007193762));
#272324=CARTESIAN_POINT('Ctrl Pts',(2.38043097016002,44.4848900869505,6.64210493853095));
#272325=CARTESIAN_POINT('Ctrl Pts',(2.40398237976074,44.0213088106809,6.38581235296264));
#272326=CARTESIAN_POINT('Ctrl Pts',(2.41030970876281,43.7479067476922,6.20244587788006));
#272327=CARTESIAN_POINT('Ctrl Pts',(2.41030970876281,43.4921152187147,5.997420928736));
#272328=CARTESIAN_POINT('',(0.0328697087628034,51.7731096363835,11.3431628416274));
#272329=CARTESIAN_POINT('Ctrl Pts',(0.0328697087628105,51.7731096363835,
11.3431628416274));
#272330=CARTESIAN_POINT('Ctrl Pts',(0.035279037872097,51.769469557838,11.3397150868991));
#272331=CARTESIAN_POINT('Ctrl Pts',(0.037686765049985,51.7658279378758,
11.3362680987956));
#272332=CARTESIAN_POINT('Ctrl Pts',(0.986850403300099,50.3286803449892,
9.97680961700231));
#272333=CARTESIAN_POINT('Ctrl Pts',(1.68188687638375,48.6641027521173,8.75189581712803));
#272334=CARTESIAN_POINT('Ctrl Pts',(2.20268963592813,46.1743002947838,7.40735308404252));
#272335=CARTESIAN_POINT('Ctrl Pts',(2.29806251068019,45.5166694401474,7.0912066452453));
#272336=CARTESIAN_POINT('Ctrl Pts',(2.35340786587133,44.8472209057106,6.80704260162844));
#272337=CARTESIAN_POINT('Origin',(0.0328697087628034,3.06591104035337,1.49207703394933));
#272338=CARTESIAN_POINT('Origin',(-16.4313702912372,3.06591104035337,1.49207703394933));
#272339=CARTESIAN_POINT('',(-6.8539302912372,51.7731096363835,11.3431628416274));
#272340=CARTESIAN_POINT('',(-3.4105302912372,51.7731096363835,11.3431628416274));
#272341=CARTESIAN_POINT('Origin',(-6.8539302912372,3.06591104035337,1.49207703394933));
#272342=CARTESIAN_POINT('Origin',(9.0566297087628,3.06591104035337,1.49207703394933));
#272343=CARTESIAN_POINT('',(-9.2313702912372,41.8295746888953,13.8190591635528));
#272344=CARTESIAN_POINT('Ctrl Pts',(-9.17446844834573,43.3968281352696,
13.6306041000145));
#272345=CARTESIAN_POINT('Ctrl Pts',(-9.21458398225972,42.8697726227144,
13.6214043118221));
#272346=CARTESIAN_POINT('Ctrl Pts',(-9.2313702912372,42.3425950372429,13.6843437823865));
#272347=CARTESIAN_POINT('Ctrl Pts',(-9.2313702912372,41.8295746888953,13.8190591635527));
#272348=CARTESIAN_POINT('',(-9.17446844834455,44.8472209057105,6.80704260162841));
#272349=CARTESIAN_POINT('Ctrl Pts',(-9.17446844834572,44.8472209057106,
6.80704260162845));
#272350=CARTESIAN_POINT('Ctrl Pts',(-9.05318343777279,46.3142649294915,
7.42976584399426));
#272351=CARTESIAN_POINT('Ctrl Pts',(-8.74406947844719,47.6830398727272,
8.18913732255413));
#272352=CARTESIAN_POINT('Ctrl Pts',(-7.90182428445088,49.9732357872253,
9.76083830442761));
#272353=CARTESIAN_POINT('Ctrl Pts',(-7.41851411808578,50.9201213637075,
10.5352422669585));
#272354=CARTESIAN_POINT('Ctrl Pts',(-6.85393029123721,51.7731096363835,
11.3431628416274));
#272355=CARTESIAN_POINT('',(-9.2313702912372,43.4921152187147,5.99742092873599));
#272356=CARTESIAN_POINT('Ctrl Pts',(-9.2313702912372,43.4921152187147,5.99742092873599));
#272357=CARTESIAN_POINT('Ctrl Pts',(-9.2313702912372,43.5930832996569,6.07835001869884));
#272358=CARTESIAN_POINT('Ctrl Pts',(-9.2303894871794,43.6968764586866,6.15596890439157));
#272359=CARTESIAN_POINT('Ctrl Pts',(-9.22181693596822,44.1319110817587,
6.45896125327636));
#272360=CARTESIAN_POINT('Ctrl Pts',(-9.20467998252585,44.4817870366871,
6.65192512723797));
#272361=CARTESIAN_POINT('Ctrl Pts',(-9.17446844834572,44.8472209057106,
6.80704260162845));
#272362=CARTESIAN_POINT('Origin',(-9.2313702912372,3.06591104035337,1.49207703394933));
#272363=CARTESIAN_POINT('Origin',(-9.2313702912372,3.06591104035337,1.49207703394933));
#272364=CARTESIAN_POINT('Origin',(-9.2313702912372,-1.53724850217529,45.2882145624979));
#272365=CARTESIAN_POINT('Origin',(-9.2313702912372,16.6742095075201,43.374113195316));
#272366=CARTESIAN_POINT('Origin',(-9.2313702912372,32.5326690847319,34.21822728948));
#272367=CARTESIAN_POINT('Origin',(-9.2313702912372,43.2960584989777,19.4036926967212));
#272368=CARTESIAN_POINT('Origin',(-9.2313702912372,47.1032899382114,1.49207703394933));
#272369=CARTESIAN_POINT('Origin',(-9.2313702912372,-40.009145471192,-7.66380887188698));
#272370=CARTESIAN_POINT('Origin',(-9.2313702912372,-40.0091454711921,10.647962939785));
#272371=CARTESIAN_POINT('Origin',(-9.2313702912372,-32.5610768757426,27.3765988997259));
#272372=CARTESIAN_POINT('Origin',(-9.2313702912372,-18.9527784085759,39.6295658755751));
#272373=CARTESIAN_POINT('Origin',(2.4103097087628,35.7335955070929,28.2773985581935));
#272374=CARTESIAN_POINT('',(2.4103097087628,44.8472209057105,6.80704260162841));
#272375=CARTESIAN_POINT('Origin',(2.4103097087628,35.7335955070929,-25.2932444902948));
#272376=CARTESIAN_POINT('',(2.4103097087628,44.8472209057105,-3.82288853372976));
#272377=CARTESIAN_POINT('Origin',(2.4103097087628,47.1032899382114,1.49207703394933));
#272378=CARTESIAN_POINT('Origin',(2.4103097087628,22.0147540361679,39.2488301609802));
#272379=CARTESIAN_POINT('',(2.4103097087628,39.0732456291471,23.3415294037746));
#272380=CARTESIAN_POINT('Origin',(2.4103097087628,43.2960584989777,19.4036926967212));
#272381=CARTESIAN_POINT('Origin',(2.4103097087628,26.2897969148727,-33.7964789362641));
#272382=CARTESIAN_POINT('Origin',(2.4103097087628,-26.9873805458071,-28.1968219421462));
#272383=CARTESIAN_POINT('Origin',(2.4103097087628,38.6351352841478,-21.2996175996284));
#272384=CARTESIAN_POINT('Origin',(2.4103097087628,-12.3135738692384,-37.8538567012059));
#272385=CARTESIAN_POINT('Origin',(2.4103097087628,43.8038975571219,12.6745415268586));
#272386=CARTESIAN_POINT('Origin',(2.4103097087628,22.0147540361684,-36.2646760930813));
#272387=CARTESIAN_POINT('Origin',(2.4103097087628,44.830231645413,-4.86186520480143));
#272388=CARTESIAN_POINT('Origin',(2.4103097087628,5.01948546643284,-40.7076220708708));
#272389=CARTESIAN_POINT('Origin',(2.4103097087628,-23.3189246551137,-31.4999144624547));
#272390=CARTESIAN_POINT('',(2.4103097087628,-36.697333482147,-12.3935665627462));
#272391=CARTESIAN_POINT('Origin',(2.4103097087628,-34.4568876295199,20.9000815051911));
#272392=CARTESIAN_POINT('',(2.4103097087628,-38.9074204377757,-1.99592492673002));
#272393=CARTESIAN_POINT('Origin',(2.4103097087628,-40.009145471192,-7.66380887188698));
#272394=CARTESIAN_POINT('Origin',(2.4103097087628,9.92883769551353,-40.1916283591834));
#272395=CARTESIAN_POINT('Origin',(2.4103097087628,-36.4647000815458,-13.4063068349397));
#272396=CARTESIAN_POINT('Origin',(2.4103097087628,-7.6187838902542,-39.3792864350547));
#272397=CARTESIAN_POINT('Origin',(2.4103097087628,-39.1068178299802,3.96027419076616));
#272398=CARTESIAN_POINT('Origin',(2.4103097087628,-36.464700081546,16.3904609028378));
#272399=CARTESIAN_POINT('',(2.4103097087628,-22.427639094175,35.0182699968983));
#272400=CARTESIAN_POINT('Origin',(2.4103097087628,9.92883769551295,43.1757824270821));
#272401=CARTESIAN_POINT('',(2.4103097087628,-13.2218486904757,40.3332355645775));
#272402=CARTESIAN_POINT('Origin',(2.4103097087628,-18.9527784085759,39.6295658755751));
#272403=CARTESIAN_POINT('Origin',(2.4103097087628,-34.4568876295197,-17.915927437293));
#272404=CARTESIAN_POINT('',(2.4103097087628,-38.9074204377757,4.98007899462811));
#272405=CARTESIAN_POINT('Origin',(2.4103097087628,-23.3189246551142,34.484068530353));
#272406=CARTESIAN_POINT('',(2.4103097087628,-36.6973334821472,15.3777206306443));
#272407=CARTESIAN_POINT('Origin',(2.4103097087628,-40.0091454711921,10.647962939785));
#272408=CARTESIAN_POINT('Origin',(2.4103097087628,-7.61878389025475,42.3634405029532));
#272409=CARTESIAN_POINT('',(2.4103097087628,-27.6118203108423,30.3504122630382));
#272410=CARTESIAN_POINT('Origin',(2.4103097087628,-32.5610768757426,27.3765988997259));
#272411=CARTESIAN_POINT('Origin',(2.4103097087628,5.01948546643226,43.6917761387695));
#272412=CARTESIAN_POINT('',(2.4103097087628,27.0732750858158,36.0980473951347));
#272413=CARTESIAN_POINT('Origin',(2.4103097087628,44.8302316454129,7.84601927270067));
#272414=CARTESIAN_POINT('',(2.4103097087628,34.9728534042383,28.9852351289796));
#272415=CARTESIAN_POINT('Origin',(2.4103097087628,32.5326690847319,34.21822728948));
#272416=CARTESIAN_POINT('Origin',(2.4103097087628,-12.3135738692389,40.8380107691044));
#272417=CARTESIAN_POINT('',(2.4103097087628,10.9222131989687,42.8708787256748));
#272418=CARTESIAN_POINT('Origin',(2.4103097087628,38.6351352841475,24.2837716675275));
#272419=CARTESIAN_POINT('',(2.4103097087628,21.0318784730198,39.5860493558137));
#272420=CARTESIAN_POINT('Origin',(2.4103097087628,16.6742095075201,43.374113195316));
#272421=CARTESIAN_POINT('Origin',(2.4103097087628,-26.9873805458075,31.1809760100444));
#272422=CARTESIAN_POINT('',(2.4103097087628,-6.58727470336753,42.4889393291034));
#272423=CARTESIAN_POINT('Origin',(2.4103097087628,26.2897969148722,36.7806330041631));
#272424=CARTESIAN_POINT('',(2.4103097087628,3.9844245570031,43.6000696953234));
#272425=CARTESIAN_POINT('Origin',(2.4103097087628,-1.53724850217529,45.2882145624979));
#272426=CARTESIAN_POINT('Origin',(15.9689897087628,20.5619110403534,5.81207703394933));
#272427=CARTESIAN_POINT('',(15.9689897087628,20.5619110403534,5.81207703394933));
#272428=CARTESIAN_POINT('',(15.9689897087628,20.5619110403534,-2.82792296605067));
#272429=CARTESIAN_POINT('Origin',(15.9689897087628,20.5619110403534,-2.82792296605067));
#272430=CARTESIAN_POINT('Origin',(15.9689897087628,3.06591104035337,5.81207703394933));
#272431=CARTESIAN_POINT('Origin',(-53.7090169915742,3.06591104035337,1.49207703394933));
#272432=CARTESIAN_POINT('',(-9.2313702912372,3.06591104035337,11.6120770339493));
#272433=CARTESIAN_POINT('Origin',(-9.2313702912372,3.06591104035337,1.49207703394933));
#272434=CARTESIAN_POINT('',(2.4103097087628,3.06591104035337,11.6120770339493));
#272435=CARTESIAN_POINT('',(-53.7090169915742,3.06591104035337,11.6120770339493));
#272436=CARTESIAN_POINT('Origin',(2.4103097087628,3.06591104035337,1.49207703394933));
#272437=CARTESIAN_POINT('Origin',(-53.7090169915742,3.06591104035337,1.49207703394933));
#272438=CARTESIAN_POINT('',(-9.2313702912372,17.555631534552,-2.82792296605067));
#272439=CARTESIAN_POINT('',(-9.2313702912372,17.555631534552,5.81207703394933));
#272440=CARTESIAN_POINT('Origin',(-9.2313702912372,3.06591104035337,1.49207703394933));
#272441=CARTESIAN_POINT('',(2.4103097087628,17.555631534552,-2.82792296605067));
#272442=CARTESIAN_POINT('',(-53.7090169915742,17.555631534552,-2.82792296605067));
#272443=CARTESIAN_POINT('',(2.4103097087628,17.555631534552,5.81207703394933));
#272444=CARTESIAN_POINT('Origin',(2.4103097087628,3.06591104035337,1.49207703394933));
#272445=CARTESIAN_POINT('',(-53.7090169915742,17.555631534552,5.81207703394933));
#272446=CARTESIAN_POINT('Origin',(-53.7090169915742,17.555631534552,-2.82792296605067));
#272447=CARTESIAN_POINT('',(-9.2313702912372,20.5619110403534,-2.82792296605067));
#272448=CARTESIAN_POINT('',(-9.2313702912372,17.555631534552,-2.82792296605067));
#272449=CARTESIAN_POINT('',(2.4103097087628,20.5619110403534,-2.82792296605067));
#272450=CARTESIAN_POINT('',(-53.7090169915742,20.5619110403534,-2.82792296605067));
#272451=CARTESIAN_POINT('',(2.4103097087628,17.555631534552,-2.82792296605067));
#272452=CARTESIAN_POINT('Origin',(-53.7090169915742,20.5619110403534,-2.82792296605067));
#272453=CARTESIAN_POINT('',(-9.2313702912372,20.5619110403534,5.81207703394933));
#272454=CARTESIAN_POINT('',(-9.2313702912372,20.5619110403534,-2.82792296605067));
#272455=CARTESIAN_POINT('',(2.4103097087628,20.5619110403534,5.81207703394933));
#272456=CARTESIAN_POINT('',(-53.7090169915742,20.5619110403534,5.81207703394933));
#272457=CARTESIAN_POINT('',(2.4103097087628,20.5619110403534,-2.82792296605067));
#272458=CARTESIAN_POINT('Origin',(-53.7090169915742,20.5619110403534,5.81207703394933));
#272459=CARTESIAN_POINT('',(-9.2313702912372,20.5619110403534,5.81207703394933));
#272460=CARTESIAN_POINT('',(2.4103097087628,20.5619110403534,5.81207703394933));
#272461=CARTESIAN_POINT('Origin',(2.4103097087628,3.06591104035337,1.49207703394933));
#272462=CARTESIAN_POINT('Origin',(-9.2313702912372,3.06591104035337,1.49207703394933));
#310586=UNCERTAINTY_MEASURE_WITH_UNIT(LENGTH_MEASURE(0.01),#310624,
'DISTANCE_ACCURACY_VALUE',
'Maximum model space distance between geometric entities at asserted c
onnectivities');
#310601=UNCERTAINTY_MEASURE_WITH_UNIT(LENGTH_MEASURE(0.01),#310624,
'DISTANCE_ACCURACY_VALUE',
'Maximum model space distance between geometric entities at asserted c
onnectivities');
#310608=(
GEOMETRIC_REPRESENTATION_CONTEXT(3)
GLOBAL_UNCERTAINTY_ASSIGNED_CONTEXT((#310586))
GLOBAL_UNIT_ASSIGNED_CONTEXT((#310624,#310626,#310627))
REPRESENTATION_CONTEXT('','3D')
);
#310623=(
GEOMETRIC_REPRESENTATION_CONTEXT(3)
GLOBAL_UNCERTAINTY_ASSIGNED_CONTEXT((#310601))
GLOBAL_UNIT_ASSIGNED_CONTEXT((#310624,#310626,#310627))
REPRESENTATION_CONTEXT('','3D')
);
#310624=(
LENGTH_UNIT()
NAMED_UNIT(*)
SI_UNIT(.MILLI.,.METRE.)
);
#310626=(
NAMED_UNIT(*)
PLANE_ANGLE_UNIT()
SI_UNIT($,.RADIAN.)
);
#310627=(
NAMED_UNIT(*)
SI_UNIT($,.STERADIAN.)
SOLID_ANGLE_UNIT()
);
#310634=SHAPE_DEFINITION_REPRESENTATION(#310655,#310899);
#310655=PRODUCT_DEFINITION_SHAPE('',$,#310921);
#310899=SHAPE_REPRESENTATION('',(#103340),#310608);
#310914=PRODUCT_DEFINITION_CONTEXT('part definition',#310979,'design');
#310921=PRODUCT_DEFINITION('15-Tooth Sprocket','15-Tooth Sprocket',#310942,
#310914);
#310942=PRODUCT_DEFINITION_FORMATION('',$,#310987);
#310979=APPLICATION_CONTEXT(
'Core Data for Automotive Mechanical Design Process');
#310980=PRODUCT_CONTEXT('part definition',#310979,'mechanical');
#310987=PRODUCT('15-Tooth Sprocket','15-Tooth Sprocket',$,(#310980));
#311003=PRESENTATION_STYLE_ASSIGNMENT((#311010));
#311010=SURFACE_STYLE_USAGE(.BOTH.,#311017);
#311017=SURFACE_SIDE_STYLE('',(#311024));
#311024=SURFACE_STYLE_FILL_AREA(#311031);
#311031=FILL_AREA_STYLE('Opaque(97,158,199)',(#311038));
#311038=FILL_AREA_STYLE_COLOUR('Opaque(97,158,199)',#311045);
#311045=COLOUR_RGB('Opaque(97,158,199)',0.380392156862745,0.619607843137255,
0.780392156862745);
ENDSEC;
END-ISO-10303-21;
